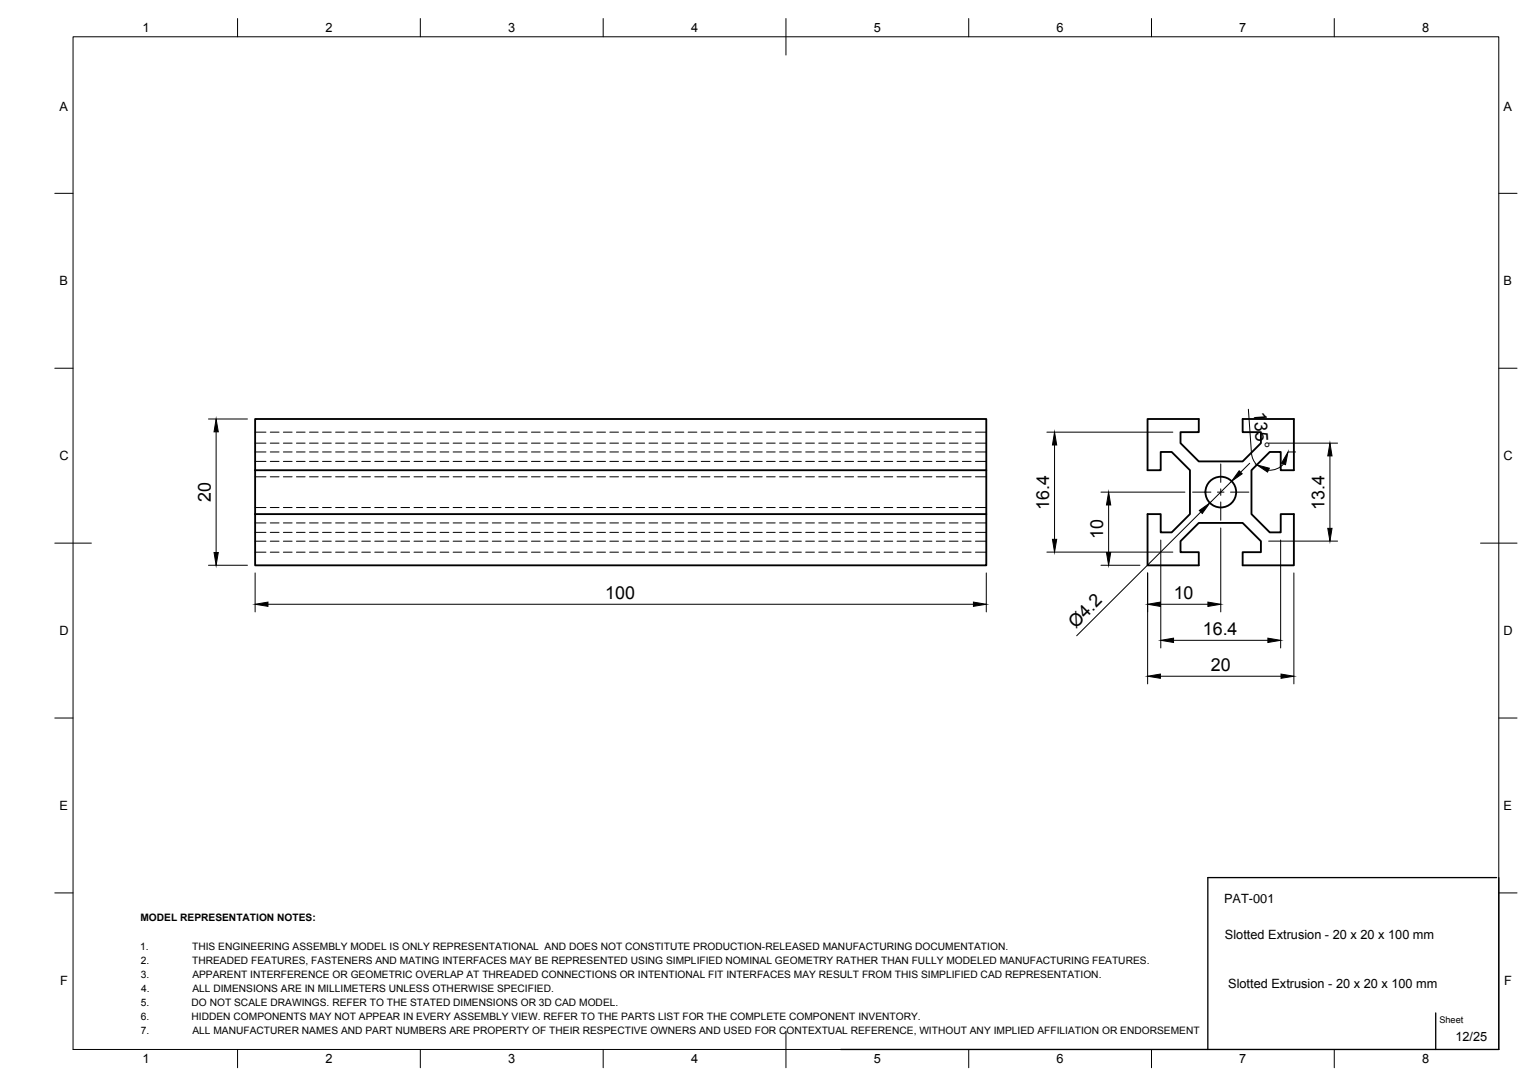
ISO-10303-21;
HEADER;
/* Generated by software containing ST-Developer
 * from STEP Tools, Inc. (www.steptools.com) 
 */

FILE_DESCRIPTION(
/* description */ ('PAT-001'),
/* implementation_level */ '2;1');

FILE_NAME(
/* name */ 'Slotted Extrusion - 20 x 20 x 100 mm.step',
/* time_stamp */ '2026-10-29T17:07:15-07:00',
/* author */ (''),
/* organization */ (''),
/* preprocessor_version */ 'ST-DEVELOPER v20.2',
/* originating_system */ 'Autodesk Translation Framework v15.17.0.0',
/* authorisation */ '');

FILE_SCHEMA (('AUTOMOTIVE_DESIGN { 1 0 10303 214 3 1 1 }'));
ENDSEC;

DATA;
#10=MECHANICAL_DESIGN_GEOMETRIC_PRESENTATION_REPRESENTATION('',(#395),#9622);
#337=SHAPE_REPRESENTATION_RELATIONSHIP('SRR','None',#9761,#362);
#362=ADVANCED_BREP_SHAPE_REPRESENTATION('',(#428),#9610);
#395=STYLED_ITEM('',(#9976),#428);
#428=MANIFOLD_SOLID_BREP('Body1',#5220);
#484=FACE_BOUND('',#1250,.T.);
#485=FACE_BOUND('',#1252,.T.);
#609=PLANE('',#5812);
#610=PLANE('',#5813);
#611=PLANE('',#5814);
#612=PLANE('',#5815);
#613=PLANE('',#5816);
#614=PLANE('',#5817);
#615=PLANE('',#5818);
#616=PLANE('',#5819);
#617=PLANE('',#5820);
#618=PLANE('',#5821);
#619=PLANE('',#5822);
#620=PLANE('',#5823);
#621=PLANE('',#5824);
#622=PLANE('',#5825);
#623=PLANE('',#5826);
#624=PLANE('',#5827);
#625=PLANE('',#5828);
#626=PLANE('',#5829);
#627=PLANE('',#5830);
#628=PLANE('',#5831);
#629=PLANE('',#5832);
#630=PLANE('',#5833);
#631=PLANE('',#5834);
#632=PLANE('',#5835);
#633=PLANE('',#5836);
#634=PLANE('',#5837);
#635=PLANE('',#5838);
#636=PLANE('',#5839);
#637=PLANE('',#5840);
#638=PLANE('',#5841);
#639=PLANE('',#5842);
#640=PLANE('',#5843);
#641=PLANE('',#5844);
#642=PLANE('',#5845);
#643=PLANE('',#5846);
#644=PLANE('',#5847);
#645=PLANE('',#5851);
#646=PLANE('',#5852);
#647=PLANE('',#5853);
#648=PLANE('',#5854);
#649=PLANE('',#5855);
#650=PLANE('',#5856);
#651=PLANE('',#5857);
#652=PLANE('',#5858);
#653=PLANE('',#5859);
#654=PLANE('',#5860);
#861=FACE_OUTER_BOUND('',#1204,.T.);
#862=FACE_OUTER_BOUND('',#1205,.T.);
#863=FACE_OUTER_BOUND('',#1206,.T.);
#864=FACE_OUTER_BOUND('',#1207,.T.);
#865=FACE_OUTER_BOUND('',#1208,.T.);
#866=FACE_OUTER_BOUND('',#1209,.T.);
#867=FACE_OUTER_BOUND('',#1210,.T.);
#868=FACE_OUTER_BOUND('',#1211,.T.);
#869=FACE_OUTER_BOUND('',#1212,.T.);
#870=FACE_OUTER_BOUND('',#1213,.T.);
#871=FACE_OUTER_BOUND('',#1214,.T.);
#872=FACE_OUTER_BOUND('',#1215,.T.);
#873=FACE_OUTER_BOUND('',#1216,.T.);
#874=FACE_OUTER_BOUND('',#1217,.T.);
#875=FACE_OUTER_BOUND('',#1218,.T.);
#876=FACE_OUTER_BOUND('',#1219,.T.);
#877=FACE_OUTER_BOUND('',#1220,.T.);
#878=FACE_OUTER_BOUND('',#1221,.T.);
#879=FACE_OUTER_BOUND('',#1222,.T.);
#880=FACE_OUTER_BOUND('',#1223,.T.);
#881=FACE_OUTER_BOUND('',#1224,.T.);
#882=FACE_OUTER_BOUND('',#1225,.T.);
#883=FACE_OUTER_BOUND('',#1226,.T.);
#884=FACE_OUTER_BOUND('',#1227,.T.);
#885=FACE_OUTER_BOUND('',#1228,.T.);
#886=FACE_OUTER_BOUND('',#1229,.T.);
#887=FACE_OUTER_BOUND('',#1230,.T.);
#888=FACE_OUTER_BOUND('',#1231,.T.);
#889=FACE_OUTER_BOUND('',#1232,.T.);
#890=FACE_OUTER_BOUND('',#1233,.T.);
#891=FACE_OUTER_BOUND('',#1234,.T.);
#892=FACE_OUTER_BOUND('',#1235,.T.);
#893=FACE_OUTER_BOUND('',#1236,.T.);
#894=FACE_OUTER_BOUND('',#1237,.T.);
#895=FACE_OUTER_BOUND('',#1238,.T.);
#896=FACE_OUTER_BOUND('',#1239,.T.);
#897=FACE_OUTER_BOUND('',#1240,.T.);
#898=FACE_OUTER_BOUND('',#1241,.T.);
#899=FACE_OUTER_BOUND('',#1242,.T.);
#900=FACE_OUTER_BOUND('',#1243,.T.);
#901=FACE_OUTER_BOUND('',#1244,.T.);
#902=FACE_OUTER_BOUND('',#1245,.T.);
#903=FACE_OUTER_BOUND('',#1246,.T.);
#904=FACE_OUTER_BOUND('',#1247,.T.);
#905=FACE_OUTER_BOUND('',#1248,.T.);
#906=FACE_OUTER_BOUND('',#1249,.T.);
#907=FACE_OUTER_BOUND('',#1251,.T.);
#1204=EDGE_LOOP('',(#4131,#4132,#4133,#4134));
#1205=EDGE_LOOP('',(#4135,#4136,#4137,#4138));
#1206=EDGE_LOOP('',(#4139,#4140,#4141,#4142));
#1207=EDGE_LOOP('',(#4143,#4144,#4145,#4146));
#1208=EDGE_LOOP('',(#4147,#4148,#4149,#4150));
#1209=EDGE_LOOP('',(#4151,#4152,#4153,#4154));
#1210=EDGE_LOOP('',(#4155,#4156,#4157,#4158));
#1211=EDGE_LOOP('',(#4159,#4160,#4161,#4162));
#1212=EDGE_LOOP('',(#4163,#4164,#4165,#4166));
#1213=EDGE_LOOP('',(#4167,#4168,#4169,#4170));
#1214=EDGE_LOOP('',(#4171,#4172,#4173,#4174));
#1215=EDGE_LOOP('',(#4175,#4176,#4177,#4178));
#1216=EDGE_LOOP('',(#4179,#4180,#4181,#4182));
#1217=EDGE_LOOP('',(#4183,#4184,#4185,#4186));
#1218=EDGE_LOOP('',(#4187,#4188,#4189,#4190));
#1219=EDGE_LOOP('',(#4191,#4192,#4193,#4194));
#1220=EDGE_LOOP('',(#4195,#4196,#4197,#4198));
#1221=EDGE_LOOP('',(#4199,#4200,#4201,#4202));
#1222=EDGE_LOOP('',(#4203,#4204,#4205,#4206));
#1223=EDGE_LOOP('',(#4207,#4208,#4209,#4210));
#1224=EDGE_LOOP('',(#4211,#4212,#4213,#4214));
#1225=EDGE_LOOP('',(#4215,#4216,#4217,#4218));
#1226=EDGE_LOOP('',(#4219,#4220,#4221,#4222));
#1227=EDGE_LOOP('',(#4223,#4224,#4225,#4226));
#1228=EDGE_LOOP('',(#4227,#4228,#4229,#4230));
#1229=EDGE_LOOP('',(#4231,#4232,#4233,#4234));
#1230=EDGE_LOOP('',(#4235,#4236,#4237,#4238));
#1231=EDGE_LOOP('',(#4239,#4240,#4241,#4242));
#1232=EDGE_LOOP('',(#4243,#4244,#4245,#4246));
#1233=EDGE_LOOP('',(#4247,#4248,#4249,#4250));
#1234=EDGE_LOOP('',(#4251,#4252,#4253,#4254));
#1235=EDGE_LOOP('',(#4255,#4256,#4257,#4258));
#1236=EDGE_LOOP('',(#4259,#4260,#4261,#4262));
#1237=EDGE_LOOP('',(#4263,#4264,#4265,#4266));
#1238=EDGE_LOOP('',(#4267,#4268,#4269,#4270));
#1239=EDGE_LOOP('',(#4271,#4272,#4273,#4274));
#1240=EDGE_LOOP('',(#4275,#4276,#4277,#4278));
#1241=EDGE_LOOP('',(#4279,#4280,#4281,#4282));
#1242=EDGE_LOOP('',(#4283,#4284,#4285,#4286));
#1243=EDGE_LOOP('',(#4287,#4288,#4289,#4290));
#1244=EDGE_LOOP('',(#4291,#4292,#4293,#4294));
#1245=EDGE_LOOP('',(#4295,#4296,#4297,#4298));
#1246=EDGE_LOOP('',(#4299,#4300,#4301,#4302));
#1247=EDGE_LOOP('',(#4303,#4304,#4305,#4306));
#1248=EDGE_LOOP('',(#4307,#4308,#4309,#4310));
#1249=EDGE_LOOP('',(#4311,#4312,#4313,#4314,#4315,#4316,#4317,#4318,#4319,
#4320,#4321,#4322,#4323,#4324,#4325,#4326,#4327,#4328,#4329,#4330,#4331,
#4332,#4333,#4334,#4335,#4336,#4337,#4338,#4339,#4340,#4341,#4342,#4343,
#4344,#4345,#4346,#4347,#4348,#4349,#4350,#4351,#4352,#4353,#4354));
#1250=EDGE_LOOP('',(#4355));
#1251=EDGE_LOOP('',(#4356,#4357,#4358,#4359,#4360,#4361,#4362,#4363,#4364,
#4365,#4366,#4367,#4368,#4369,#4370,#4371,#4372,#4373,#4374,#4375,#4376,
#4377,#4378,#4379,#4380,#4381,#4382,#4383,#4384,#4385,#4386,#4387,#4388,
#4389,#4390,#4391,#4392,#4393,#4394,#4395,#4396,#4397,#4398,#4399));
#1252=EDGE_LOOP('',(#4400));
#1553=LINE('',#8739,#1958);
#1554=LINE('',#8741,#1959);
#1555=LINE('',#8743,#1960);
#1556=LINE('',#8744,#1961);
#1557=LINE('',#8747,#1962);
#1558=LINE('',#8749,#1963);
#1559=LINE('',#8750,#1964);
#1560=LINE('',#8753,#1965);
#1561=LINE('',#8755,#1966);
#1562=LINE('',#8756,#1967);
#1563=LINE('',#8759,#1968);
#1564=LINE('',#8761,#1969);
#1565=LINE('',#8762,#1970);
#1566=LINE('',#8765,#1971);
#1567=LINE('',#8767,#1972);
#1568=LINE('',#8768,#1973);
#1569=LINE('',#8771,#1974);
#1570=LINE('',#8773,#1975);
#1571=LINE('',#8774,#1976);
#1572=LINE('',#8777,#1977);
#1573=LINE('',#8779,#1978);
#1574=LINE('',#8780,#1979);
#1575=LINE('',#8783,#1980);
#1576=LINE('',#8785,#1981);
#1577=LINE('',#8786,#1982);
#1578=LINE('',#8789,#1983);
#1579=LINE('',#8791,#1984);
#1580=LINE('',#8792,#1985);
#1581=LINE('',#8796,#1986);
#1582=LINE('',#8798,#1987);
#1583=LINE('',#8800,#1988);
#1584=LINE('',#8801,#1989);
#1585=LINE('',#8804,#1990);
#1586=LINE('',#8806,#1991);
#1587=LINE('',#8807,#1992);
#1588=LINE('',#8810,#1993);
#1589=LINE('',#8812,#1994);
#1590=LINE('',#8813,#1995);
#1591=LINE('',#8816,#1996);
#1592=LINE('',#8818,#1997);
#1593=LINE('',#8819,#1998);
#1594=LINE('',#8822,#1999);
#1595=LINE('',#8824,#2000);
#1596=LINE('',#8825,#2001);
#1597=LINE('',#8828,#2002);
#1598=LINE('',#8830,#2003);
#1599=LINE('',#8831,#2004);
#1600=LINE('',#8834,#2005);
#1601=LINE('',#8836,#2006);
#1602=LINE('',#8837,#2007);
#1603=LINE('',#8840,#2008);
#1604=LINE('',#8842,#2009);
#1605=LINE('',#8843,#2010);
#1606=LINE('',#8846,#2011);
#1607=LINE('',#8848,#2012);
#1608=LINE('',#8849,#2013);
#1609=LINE('',#8853,#2014);
#1610=LINE('',#8855,#2015);
#1611=LINE('',#8857,#2016);
#1612=LINE('',#8858,#2017);
#1613=LINE('',#8861,#2018);
#1614=LINE('',#8863,#2019);
#1615=LINE('',#8864,#2020);
#1616=LINE('',#8867,#2021);
#1617=LINE('',#8869,#2022);
#1618=LINE('',#8870,#2023);
#1619=LINE('',#8873,#2024);
#1620=LINE('',#8875,#2025);
#1621=LINE('',#8876,#2026);
#1622=LINE('',#8879,#2027);
#1623=LINE('',#8881,#2028);
#1624=LINE('',#8882,#2029);
#1625=LINE('',#8885,#2030);
#1626=LINE('',#8887,#2031);
#1627=LINE('',#8888,#2032);
#1628=LINE('',#8891,#2033);
#1629=LINE('',#8893,#2034);
#1630=LINE('',#8894,#2035);
#1631=LINE('',#8897,#2036);
#1632=LINE('',#8899,#2037);
#1633=LINE('',#8900,#2038);
#1634=LINE('',#8903,#2039);
#1635=LINE('',#8905,#2040);
#1636=LINE('',#8906,#2041);
#1637=LINE('',#8910,#2042);
#1638=LINE('',#8912,#2043);
#1639=LINE('',#8914,#2044);
#1640=LINE('',#8915,#2045);
#1641=LINE('',#8918,#2046);
#1642=LINE('',#8920,#2047);
#1643=LINE('',#8921,#2048);
#1644=LINE('',#8924,#2049);
#1645=LINE('',#8926,#2050);
#1646=LINE('',#8927,#2051);
#1647=LINE('',#8930,#2052);
#1648=LINE('',#8932,#2053);
#1649=LINE('',#8933,#2054);
#1650=LINE('',#8936,#2055);
#1651=LINE('',#8938,#2056);
#1652=LINE('',#8939,#2057);
#1653=LINE('',#8942,#2058);
#1654=LINE('',#8944,#2059);
#1655=LINE('',#8945,#2060);
#1656=LINE('',#8948,#2061);
#1657=LINE('',#8950,#2062);
#1658=LINE('',#8951,#2063);
#1659=LINE('',#8954,#2064);
#1660=LINE('',#8956,#2065);
#1661=LINE('',#8957,#2066);
#1662=LINE('',#8960,#2067);
#1663=LINE('',#8962,#2068);
#1664=LINE('',#8963,#2069);
#1665=LINE('',#8968,#2070);
#1666=LINE('',#8972,#2071);
#1667=LINE('',#8974,#2072);
#1668=LINE('',#8975,#2073);
#1669=LINE('',#8978,#2074);
#1670=LINE('',#8980,#2075);
#1671=LINE('',#8981,#2076);
#1672=LINE('',#8983,#2077);
#1673=LINE('',#8984,#2078);
#1674=LINE('',#8987,#2079);
#1675=LINE('',#8989,#2080);
#1676=LINE('',#8990,#2081);
#1677=LINE('',#8992,#2082);
#1678=LINE('',#8993,#2083);
#1679=LINE('',#8996,#2084);
#1680=LINE('',#8998,#2085);
#1681=LINE('',#8999,#2086);
#1682=LINE('',#9001,#2087);
#1683=LINE('',#9002,#2088);
#1684=LINE('',#9004,#2089);
#1685=LINE('',#9005,#2090);
#1958=VECTOR('',#6870,1.);
#1959=VECTOR('',#6871,1.);
#1960=VECTOR('',#6872,1.);
#1961=VECTOR('',#6873,1.);
#1962=VECTOR('',#6876,1.);
#1963=VECTOR('',#6877,1.);
#1964=VECTOR('',#6878,1.);
#1965=VECTOR('',#6881,1.);
#1966=VECTOR('',#6882,1.);
#1967=VECTOR('',#6883,1.);
#1968=VECTOR('',#6886,1.);
#1969=VECTOR('',#6887,1.);
#1970=VECTOR('',#6888,1.);
#1971=VECTOR('',#6891,1.);
#1972=VECTOR('',#6892,1.);
#1973=VECTOR('',#6893,1.);
#1974=VECTOR('',#6896,1.);
#1975=VECTOR('',#6897,1.);
#1976=VECTOR('',#6898,1.);
#1977=VECTOR('',#6901,1.);
#1978=VECTOR('',#6902,1.);
#1979=VECTOR('',#6903,1.);
#1980=VECTOR('',#6906,1.);
#1981=VECTOR('',#6907,1.);
#1982=VECTOR('',#6908,1.);
#1983=VECTOR('',#6911,1.);
#1984=VECTOR('',#6912,1.);
#1985=VECTOR('',#6913,1.);
#1986=VECTOR('',#6916,1.);
#1987=VECTOR('',#6917,1.);
#1988=VECTOR('',#6918,1.);
#1989=VECTOR('',#6919,1.);
#1990=VECTOR('',#6922,1.);
#1991=VECTOR('',#6923,1.);
#1992=VECTOR('',#6924,1.);
#1993=VECTOR('',#6927,1.);
#1994=VECTOR('',#6928,1.);
#1995=VECTOR('',#6929,1.);
#1996=VECTOR('',#6932,1.);
#1997=VECTOR('',#6933,1.);
#1998=VECTOR('',#6934,1.);
#1999=VECTOR('',#6937,1.);
#2000=VECTOR('',#6938,1.);
#2001=VECTOR('',#6939,1.);
#2002=VECTOR('',#6942,1.);
#2003=VECTOR('',#6943,1.);
#2004=VECTOR('',#6944,1.);
#2005=VECTOR('',#6947,1.);
#2006=VECTOR('',#6948,1.);
#2007=VECTOR('',#6949,1.);
#2008=VECTOR('',#6952,1.);
#2009=VECTOR('',#6953,1.);
#2010=VECTOR('',#6954,1.);
#2011=VECTOR('',#6957,1.);
#2012=VECTOR('',#6958,1.);
#2013=VECTOR('',#6959,1.);
#2014=VECTOR('',#6962,1.);
#2015=VECTOR('',#6963,1.);
#2016=VECTOR('',#6964,1.);
#2017=VECTOR('',#6965,1.);
#2018=VECTOR('',#6968,1.);
#2019=VECTOR('',#6969,1.);
#2020=VECTOR('',#6970,1.);
#2021=VECTOR('',#6973,1.);
#2022=VECTOR('',#6974,1.);
#2023=VECTOR('',#6975,1.);
#2024=VECTOR('',#6978,1.);
#2025=VECTOR('',#6979,1.);
#2026=VECTOR('',#6980,1.);
#2027=VECTOR('',#6983,1.);
#2028=VECTOR('',#6984,1.);
#2029=VECTOR('',#6985,1.);
#2030=VECTOR('',#6988,1.);
#2031=VECTOR('',#6989,1.);
#2032=VECTOR('',#6990,1.);
#2033=VECTOR('',#6993,1.);
#2034=VECTOR('',#6994,1.);
#2035=VECTOR('',#6995,1.);
#2036=VECTOR('',#6998,1.);
#2037=VECTOR('',#6999,1.);
#2038=VECTOR('',#7000,1.);
#2039=VECTOR('',#7003,1.);
#2040=VECTOR('',#7004,1.);
#2041=VECTOR('',#7005,1.);
#2042=VECTOR('',#7008,1.);
#2043=VECTOR('',#7009,1.);
#2044=VECTOR('',#7010,1.);
#2045=VECTOR('',#7011,1.);
#2046=VECTOR('',#7014,1.);
#2047=VECTOR('',#7015,1.);
#2048=VECTOR('',#7016,1.);
#2049=VECTOR('',#7019,1.);
#2050=VECTOR('',#7020,1.);
#2051=VECTOR('',#7021,1.);
#2052=VECTOR('',#7024,1.);
#2053=VECTOR('',#7025,1.);
#2054=VECTOR('',#7026,1.);
#2055=VECTOR('',#7029,1.);
#2056=VECTOR('',#7030,1.);
#2057=VECTOR('',#7031,1.);
#2058=VECTOR('',#7034,1.);
#2059=VECTOR('',#7035,1.);
#2060=VECTOR('',#7036,1.);
#2061=VECTOR('',#7039,1.);
#2062=VECTOR('',#7040,1.);
#2063=VECTOR('',#7041,1.);
#2064=VECTOR('',#7044,1.);
#2065=VECTOR('',#7045,1.);
#2066=VECTOR('',#7046,1.);
#2067=VECTOR('',#7049,1.);
#2068=VECTOR('',#7050,1.);
#2069=VECTOR('',#7051,1.);
#2070=VECTOR('',#7056,0.21);
#2071=VECTOR('',#7061,1.);
#2072=VECTOR('',#7062,1.);
#2073=VECTOR('',#7063,1.);
#2074=VECTOR('',#7066,1.);
#2075=VECTOR('',#7067,1.);
#2076=VECTOR('',#7068,1.);
#2077=VECTOR('',#7071,1.);
#2078=VECTOR('',#7072,1.);
#2079=VECTOR('',#7075,1.);
#2080=VECTOR('',#7076,1.);
#2081=VECTOR('',#7077,1.);
#2082=VECTOR('',#7080,1.);
#2083=VECTOR('',#7081,1.);
#2084=VECTOR('',#7084,1.);
#2085=VECTOR('',#7085,1.);
#2086=VECTOR('',#7086,1.);
#2087=VECTOR('',#7089,1.);
#2088=VECTOR('',#7090,1.);
#2089=VECTOR('',#7093,1.);
#2090=VECTOR('',#7094,1.);
#2342=CIRCLE('',#5849,0.21);
#2343=CIRCLE('',#5850,0.21);
#2634=VERTEX_POINT('',#8737);
#2635=VERTEX_POINT('',#8738);
#2636=VERTEX_POINT('',#8740);
#2637=VERTEX_POINT('',#8742);
#2638=VERTEX_POINT('',#8746);
#2639=VERTEX_POINT('',#8748);
#2640=VERTEX_POINT('',#8752);
#2641=VERTEX_POINT('',#8754);
#2642=VERTEX_POINT('',#8758);
#2643=VERTEX_POINT('',#8760);
#2644=VERTEX_POINT('',#8764);
#2645=VERTEX_POINT('',#8766);
#2646=VERTEX_POINT('',#8770);
#2647=VERTEX_POINT('',#8772);
#2648=VERTEX_POINT('',#8776);
#2649=VERTEX_POINT('',#8778);
#2650=VERTEX_POINT('',#8782);
#2651=VERTEX_POINT('',#8784);
#2652=VERTEX_POINT('',#8788);
#2653=VERTEX_POINT('',#8790);
#2654=VERTEX_POINT('',#8794);
#2655=VERTEX_POINT('',#8795);
#2656=VERTEX_POINT('',#8797);
#2657=VERTEX_POINT('',#8799);
#2658=VERTEX_POINT('',#8803);
#2659=VERTEX_POINT('',#8805);
#2660=VERTEX_POINT('',#8809);
#2661=VERTEX_POINT('',#8811);
#2662=VERTEX_POINT('',#8815);
#2663=VERTEX_POINT('',#8817);
#2664=VERTEX_POINT('',#8821);
#2665=VERTEX_POINT('',#8823);
#2666=VERTEX_POINT('',#8827);
#2667=VERTEX_POINT('',#8829);
#2668=VERTEX_POINT('',#8833);
#2669=VERTEX_POINT('',#8835);
#2670=VERTEX_POINT('',#8839);
#2671=VERTEX_POINT('',#8841);
#2672=VERTEX_POINT('',#8845);
#2673=VERTEX_POINT('',#8847);
#2674=VERTEX_POINT('',#8851);
#2675=VERTEX_POINT('',#8852);
#2676=VERTEX_POINT('',#8854);
#2677=VERTEX_POINT('',#8856);
#2678=VERTEX_POINT('',#8860);
#2679=VERTEX_POINT('',#8862);
#2680=VERTEX_POINT('',#8866);
#2681=VERTEX_POINT('',#8868);
#2682=VERTEX_POINT('',#8872);
#2683=VERTEX_POINT('',#8874);
#2684=VERTEX_POINT('',#8878);
#2685=VERTEX_POINT('',#8880);
#2686=VERTEX_POINT('',#8884);
#2687=VERTEX_POINT('',#8886);
#2688=VERTEX_POINT('',#8890);
#2689=VERTEX_POINT('',#8892);
#2690=VERTEX_POINT('',#8896);
#2691=VERTEX_POINT('',#8898);
#2692=VERTEX_POINT('',#8902);
#2693=VERTEX_POINT('',#8904);
#2694=VERTEX_POINT('',#8908);
#2695=VERTEX_POINT('',#8909);
#2696=VERTEX_POINT('',#8911);
#2697=VERTEX_POINT('',#8913);
#2698=VERTEX_POINT('',#8917);
#2699=VERTEX_POINT('',#8919);
#2700=VERTEX_POINT('',#8923);
#2701=VERTEX_POINT('',#8925);
#2702=VERTEX_POINT('',#8929);
#2703=VERTEX_POINT('',#8931);
#2704=VERTEX_POINT('',#8935);
#2705=VERTEX_POINT('',#8937);
#2706=VERTEX_POINT('',#8941);
#2707=VERTEX_POINT('',#8943);
#2708=VERTEX_POINT('',#8947);
#2709=VERTEX_POINT('',#8949);
#2710=VERTEX_POINT('',#8953);
#2711=VERTEX_POINT('',#8955);
#2712=VERTEX_POINT('',#8959);
#2713=VERTEX_POINT('',#8961);
#2714=VERTEX_POINT('',#8965);
#2715=VERTEX_POINT('',#8967);
#2716=VERTEX_POINT('',#8971);
#2717=VERTEX_POINT('',#8973);
#2718=VERTEX_POINT('',#8977);
#2719=VERTEX_POINT('',#8979);
#2720=VERTEX_POINT('',#8986);
#2721=VERTEX_POINT('',#8988);
#2722=VERTEX_POINT('',#8995);
#2723=VERTEX_POINT('',#8997);
#3169=EDGE_CURVE('',#2634,#2635,#1553,.T.);
#3170=EDGE_CURVE('',#2634,#2636,#1554,.T.);
#3171=EDGE_CURVE('',#2637,#2636,#1555,.T.);
#3172=EDGE_CURVE('',#2635,#2637,#1556,.T.);
#3173=EDGE_CURVE('',#2638,#2634,#1557,.T.);
#3174=EDGE_CURVE('',#2638,#2639,#1558,.T.);
#3175=EDGE_CURVE('',#2636,#2639,#1559,.T.);
#3176=EDGE_CURVE('',#2640,#2638,#1560,.T.);
#3177=EDGE_CURVE('',#2640,#2641,#1561,.T.);
#3178=EDGE_CURVE('',#2639,#2641,#1562,.T.);
#3179=EDGE_CURVE('',#2642,#2640,#1563,.T.);
#3180=EDGE_CURVE('',#2642,#2643,#1564,.T.);
#3181=EDGE_CURVE('',#2641,#2643,#1565,.T.);
#3182=EDGE_CURVE('',#2644,#2642,#1566,.T.);
#3183=EDGE_CURVE('',#2644,#2645,#1567,.T.);
#3184=EDGE_CURVE('',#2643,#2645,#1568,.T.);
#3185=EDGE_CURVE('',#2646,#2644,#1569,.T.);
#3186=EDGE_CURVE('',#2646,#2647,#1570,.T.);
#3187=EDGE_CURVE('',#2645,#2647,#1571,.T.);
#3188=EDGE_CURVE('',#2648,#2646,#1572,.T.);
#3189=EDGE_CURVE('',#2648,#2649,#1573,.T.);
#3190=EDGE_CURVE('',#2647,#2649,#1574,.T.);
#3191=EDGE_CURVE('',#2650,#2648,#1575,.T.);
#3192=EDGE_CURVE('',#2650,#2651,#1576,.T.);
#3193=EDGE_CURVE('',#2649,#2651,#1577,.T.);
#3194=EDGE_CURVE('',#2652,#2650,#1578,.T.);
#3195=EDGE_CURVE('',#2653,#2652,#1579,.T.);
#3196=EDGE_CURVE('',#2651,#2653,#1580,.T.);
#3197=EDGE_CURVE('',#2654,#2655,#1581,.T.);
#3198=EDGE_CURVE('',#2654,#2656,#1582,.T.);
#3199=EDGE_CURVE('',#2657,#2656,#1583,.T.);
#3200=EDGE_CURVE('',#2655,#2657,#1584,.T.);
#3201=EDGE_CURVE('',#2658,#2654,#1585,.T.);
#3202=EDGE_CURVE('',#2658,#2659,#1586,.T.);
#3203=EDGE_CURVE('',#2656,#2659,#1587,.T.);
#3204=EDGE_CURVE('',#2660,#2658,#1588,.T.);
#3205=EDGE_CURVE('',#2660,#2661,#1589,.T.);
#3206=EDGE_CURVE('',#2659,#2661,#1590,.T.);
#3207=EDGE_CURVE('',#2662,#2660,#1591,.T.);
#3208=EDGE_CURVE('',#2662,#2663,#1592,.T.);
#3209=EDGE_CURVE('',#2661,#2663,#1593,.T.);
#3210=EDGE_CURVE('',#2664,#2662,#1594,.T.);
#3211=EDGE_CURVE('',#2664,#2665,#1595,.T.);
#3212=EDGE_CURVE('',#2663,#2665,#1596,.T.);
#3213=EDGE_CURVE('',#2666,#2664,#1597,.T.);
#3214=EDGE_CURVE('',#2666,#2667,#1598,.T.);
#3215=EDGE_CURVE('',#2665,#2667,#1599,.T.);
#3216=EDGE_CURVE('',#2668,#2666,#1600,.T.);
#3217=EDGE_CURVE('',#2668,#2669,#1601,.T.);
#3218=EDGE_CURVE('',#2667,#2669,#1602,.T.);
#3219=EDGE_CURVE('',#2670,#2668,#1603,.T.);
#3220=EDGE_CURVE('',#2670,#2671,#1604,.T.);
#3221=EDGE_CURVE('',#2669,#2671,#1605,.T.);
#3222=EDGE_CURVE('',#2672,#2670,#1606,.T.);
#3223=EDGE_CURVE('',#2673,#2672,#1607,.T.);
#3224=EDGE_CURVE('',#2671,#2673,#1608,.T.);
#3225=EDGE_CURVE('',#2674,#2675,#1609,.T.);
#3226=EDGE_CURVE('',#2674,#2676,#1610,.T.);
#3227=EDGE_CURVE('',#2677,#2676,#1611,.T.);
#3228=EDGE_CURVE('',#2675,#2677,#1612,.T.);
#3229=EDGE_CURVE('',#2678,#2674,#1613,.T.);
#3230=EDGE_CURVE('',#2678,#2679,#1614,.T.);
#3231=EDGE_CURVE('',#2676,#2679,#1615,.T.);
#3232=EDGE_CURVE('',#2680,#2678,#1616,.T.);
#3233=EDGE_CURVE('',#2680,#2681,#1617,.T.);
#3234=EDGE_CURVE('',#2679,#2681,#1618,.T.);
#3235=EDGE_CURVE('',#2682,#2680,#1619,.T.);
#3236=EDGE_CURVE('',#2682,#2683,#1620,.T.);
#3237=EDGE_CURVE('',#2681,#2683,#1621,.T.);
#3238=EDGE_CURVE('',#2684,#2682,#1622,.T.);
#3239=EDGE_CURVE('',#2684,#2685,#1623,.T.);
#3240=EDGE_CURVE('',#2683,#2685,#1624,.T.);
#3241=EDGE_CURVE('',#2686,#2684,#1625,.T.);
#3242=EDGE_CURVE('',#2686,#2687,#1626,.T.);
#3243=EDGE_CURVE('',#2685,#2687,#1627,.T.);
#3244=EDGE_CURVE('',#2688,#2686,#1628,.T.);
#3245=EDGE_CURVE('',#2688,#2689,#1629,.T.);
#3246=EDGE_CURVE('',#2687,#2689,#1630,.T.);
#3247=EDGE_CURVE('',#2690,#2688,#1631,.T.);
#3248=EDGE_CURVE('',#2690,#2691,#1632,.T.);
#3249=EDGE_CURVE('',#2689,#2691,#1633,.T.);
#3250=EDGE_CURVE('',#2692,#2690,#1634,.T.);
#3251=EDGE_CURVE('',#2693,#2692,#1635,.T.);
#3252=EDGE_CURVE('',#2691,#2693,#1636,.T.);
#3253=EDGE_CURVE('',#2694,#2695,#1637,.T.);
#3254=EDGE_CURVE('',#2694,#2696,#1638,.T.);
#3255=EDGE_CURVE('',#2697,#2696,#1639,.T.);
#3256=EDGE_CURVE('',#2695,#2697,#1640,.T.);
#3257=EDGE_CURVE('',#2698,#2694,#1641,.T.);
#3258=EDGE_CURVE('',#2698,#2699,#1642,.T.);
#3259=EDGE_CURVE('',#2696,#2699,#1643,.T.);
#3260=EDGE_CURVE('',#2700,#2698,#1644,.T.);
#3261=EDGE_CURVE('',#2700,#2701,#1645,.T.);
#3262=EDGE_CURVE('',#2699,#2701,#1646,.T.);
#3263=EDGE_CURVE('',#2702,#2700,#1647,.T.);
#3264=EDGE_CURVE('',#2702,#2703,#1648,.T.);
#3265=EDGE_CURVE('',#2701,#2703,#1649,.T.);
#3266=EDGE_CURVE('',#2704,#2702,#1650,.T.);
#3267=EDGE_CURVE('',#2704,#2705,#1651,.T.);
#3268=EDGE_CURVE('',#2703,#2705,#1652,.T.);
#3269=EDGE_CURVE('',#2706,#2704,#1653,.T.);
#3270=EDGE_CURVE('',#2706,#2707,#1654,.T.);
#3271=EDGE_CURVE('',#2705,#2707,#1655,.T.);
#3272=EDGE_CURVE('',#2708,#2706,#1656,.T.);
#3273=EDGE_CURVE('',#2708,#2709,#1657,.T.);
#3274=EDGE_CURVE('',#2707,#2709,#1658,.T.);
#3275=EDGE_CURVE('',#2710,#2708,#1659,.T.);
#3276=EDGE_CURVE('',#2710,#2711,#1660,.T.);
#3277=EDGE_CURVE('',#2709,#2711,#1661,.T.);
#3278=EDGE_CURVE('',#2712,#2710,#1662,.T.);
#3279=EDGE_CURVE('',#2713,#2712,#1663,.T.);
#3280=EDGE_CURVE('',#2711,#2713,#1664,.T.);
#3281=EDGE_CURVE('',#2714,#2714,#2342,.T.);
#3282=EDGE_CURVE('',#2714,#2715,#1665,.T.);
#3283=EDGE_CURVE('',#2715,#2715,#2343,.T.);
#3284=EDGE_CURVE('',#2652,#2716,#1666,.T.);
#3285=EDGE_CURVE('',#2716,#2717,#1667,.T.);
#3286=EDGE_CURVE('',#2653,#2717,#1668,.T.);
#3287=EDGE_CURVE('',#2718,#2637,#1669,.T.);
#3288=EDGE_CURVE('',#2719,#2718,#1670,.T.);
#3289=EDGE_CURVE('',#2719,#2635,#1671,.T.);
#3290=EDGE_CURVE('',#2672,#2719,#1672,.T.);
#3291=EDGE_CURVE('',#2673,#2718,#1673,.T.);
#3292=EDGE_CURVE('',#2720,#2657,#1674,.T.);
#3293=EDGE_CURVE('',#2721,#2720,#1675,.T.);
#3294=EDGE_CURVE('',#2721,#2655,#1676,.T.);
#3295=EDGE_CURVE('',#2692,#2721,#1677,.T.);
#3296=EDGE_CURVE('',#2693,#2720,#1678,.T.);
#3297=EDGE_CURVE('',#2722,#2677,#1679,.T.);
#3298=EDGE_CURVE('',#2723,#2722,#1680,.T.);
#3299=EDGE_CURVE('',#2723,#2675,#1681,.T.);
#3300=EDGE_CURVE('',#2712,#2723,#1682,.T.);
#3301=EDGE_CURVE('',#2713,#2722,#1683,.T.);
#3302=EDGE_CURVE('',#2717,#2697,#1684,.T.);
#3303=EDGE_CURVE('',#2716,#2695,#1685,.T.);
#4131=ORIENTED_EDGE('',*,*,#3169,.F.);
#4132=ORIENTED_EDGE('',*,*,#3170,.T.);
#4133=ORIENTED_EDGE('',*,*,#3171,.F.);
#4134=ORIENTED_EDGE('',*,*,#3172,.F.);
#4135=ORIENTED_EDGE('',*,*,#3173,.F.);
#4136=ORIENTED_EDGE('',*,*,#3174,.T.);
#4137=ORIENTED_EDGE('',*,*,#3175,.F.);
#4138=ORIENTED_EDGE('',*,*,#3170,.F.);
#4139=ORIENTED_EDGE('',*,*,#3176,.F.);
#4140=ORIENTED_EDGE('',*,*,#3177,.T.);
#4141=ORIENTED_EDGE('',*,*,#3178,.F.);
#4142=ORIENTED_EDGE('',*,*,#3174,.F.);
#4143=ORIENTED_EDGE('',*,*,#3179,.F.);
#4144=ORIENTED_EDGE('',*,*,#3180,.T.);
#4145=ORIENTED_EDGE('',*,*,#3181,.F.);
#4146=ORIENTED_EDGE('',*,*,#3177,.F.);
#4147=ORIENTED_EDGE('',*,*,#3182,.F.);
#4148=ORIENTED_EDGE('',*,*,#3183,.T.);
#4149=ORIENTED_EDGE('',*,*,#3184,.F.);
#4150=ORIENTED_EDGE('',*,*,#3180,.F.);
#4151=ORIENTED_EDGE('',*,*,#3185,.F.);
#4152=ORIENTED_EDGE('',*,*,#3186,.T.);
#4153=ORIENTED_EDGE('',*,*,#3187,.F.);
#4154=ORIENTED_EDGE('',*,*,#3183,.F.);
#4155=ORIENTED_EDGE('',*,*,#3188,.F.);
#4156=ORIENTED_EDGE('',*,*,#3189,.T.);
#4157=ORIENTED_EDGE('',*,*,#3190,.F.);
#4158=ORIENTED_EDGE('',*,*,#3186,.F.);
#4159=ORIENTED_EDGE('',*,*,#3191,.F.);
#4160=ORIENTED_EDGE('',*,*,#3192,.T.);
#4161=ORIENTED_EDGE('',*,*,#3193,.F.);
#4162=ORIENTED_EDGE('',*,*,#3189,.F.);
#4163=ORIENTED_EDGE('',*,*,#3194,.F.);
#4164=ORIENTED_EDGE('',*,*,#3195,.F.);
#4165=ORIENTED_EDGE('',*,*,#3196,.F.);
#4166=ORIENTED_EDGE('',*,*,#3192,.F.);
#4167=ORIENTED_EDGE('',*,*,#3197,.F.);
#4168=ORIENTED_EDGE('',*,*,#3198,.T.);
#4169=ORIENTED_EDGE('',*,*,#3199,.F.);
#4170=ORIENTED_EDGE('',*,*,#3200,.F.);
#4171=ORIENTED_EDGE('',*,*,#3201,.F.);
#4172=ORIENTED_EDGE('',*,*,#3202,.T.);
#4173=ORIENTED_EDGE('',*,*,#3203,.F.);
#4174=ORIENTED_EDGE('',*,*,#3198,.F.);
#4175=ORIENTED_EDGE('',*,*,#3204,.F.);
#4176=ORIENTED_EDGE('',*,*,#3205,.T.);
#4177=ORIENTED_EDGE('',*,*,#3206,.F.);
#4178=ORIENTED_EDGE('',*,*,#3202,.F.);
#4179=ORIENTED_EDGE('',*,*,#3207,.F.);
#4180=ORIENTED_EDGE('',*,*,#3208,.T.);
#4181=ORIENTED_EDGE('',*,*,#3209,.F.);
#4182=ORIENTED_EDGE('',*,*,#3205,.F.);
#4183=ORIENTED_EDGE('',*,*,#3210,.F.);
#4184=ORIENTED_EDGE('',*,*,#3211,.T.);
#4185=ORIENTED_EDGE('',*,*,#3212,.F.);
#4186=ORIENTED_EDGE('',*,*,#3208,.F.);
#4187=ORIENTED_EDGE('',*,*,#3213,.F.);
#4188=ORIENTED_EDGE('',*,*,#3214,.T.);
#4189=ORIENTED_EDGE('',*,*,#3215,.F.);
#4190=ORIENTED_EDGE('',*,*,#3211,.F.);
#4191=ORIENTED_EDGE('',*,*,#3216,.F.);
#4192=ORIENTED_EDGE('',*,*,#3217,.T.);
#4193=ORIENTED_EDGE('',*,*,#3218,.F.);
#4194=ORIENTED_EDGE('',*,*,#3214,.F.);
#4195=ORIENTED_EDGE('',*,*,#3219,.F.);
#4196=ORIENTED_EDGE('',*,*,#3220,.T.);
#4197=ORIENTED_EDGE('',*,*,#3221,.F.);
#4198=ORIENTED_EDGE('',*,*,#3217,.F.);
#4199=ORIENTED_EDGE('',*,*,#3222,.F.);
#4200=ORIENTED_EDGE('',*,*,#3223,.F.);
#4201=ORIENTED_EDGE('',*,*,#3224,.F.);
#4202=ORIENTED_EDGE('',*,*,#3220,.F.);
#4203=ORIENTED_EDGE('',*,*,#3225,.F.);
#4204=ORIENTED_EDGE('',*,*,#3226,.T.);
#4205=ORIENTED_EDGE('',*,*,#3227,.F.);
#4206=ORIENTED_EDGE('',*,*,#3228,.F.);
#4207=ORIENTED_EDGE('',*,*,#3229,.F.);
#4208=ORIENTED_EDGE('',*,*,#3230,.T.);
#4209=ORIENTED_EDGE('',*,*,#3231,.F.);
#4210=ORIENTED_EDGE('',*,*,#3226,.F.);
#4211=ORIENTED_EDGE('',*,*,#3232,.F.);
#4212=ORIENTED_EDGE('',*,*,#3233,.T.);
#4213=ORIENTED_EDGE('',*,*,#3234,.F.);
#4214=ORIENTED_EDGE('',*,*,#3230,.F.);
#4215=ORIENTED_EDGE('',*,*,#3235,.F.);
#4216=ORIENTED_EDGE('',*,*,#3236,.T.);
#4217=ORIENTED_EDGE('',*,*,#3237,.F.);
#4218=ORIENTED_EDGE('',*,*,#3233,.F.);
#4219=ORIENTED_EDGE('',*,*,#3238,.F.);
#4220=ORIENTED_EDGE('',*,*,#3239,.T.);
#4221=ORIENTED_EDGE('',*,*,#3240,.F.);
#4222=ORIENTED_EDGE('',*,*,#3236,.F.);
#4223=ORIENTED_EDGE('',*,*,#3241,.F.);
#4224=ORIENTED_EDGE('',*,*,#3242,.T.);
#4225=ORIENTED_EDGE('',*,*,#3243,.F.);
#4226=ORIENTED_EDGE('',*,*,#3239,.F.);
#4227=ORIENTED_EDGE('',*,*,#3244,.F.);
#4228=ORIENTED_EDGE('',*,*,#3245,.T.);
#4229=ORIENTED_EDGE('',*,*,#3246,.F.);
#4230=ORIENTED_EDGE('',*,*,#3242,.F.);
#4231=ORIENTED_EDGE('',*,*,#3247,.F.);
#4232=ORIENTED_EDGE('',*,*,#3248,.T.);
#4233=ORIENTED_EDGE('',*,*,#3249,.F.);
#4234=ORIENTED_EDGE('',*,*,#3245,.F.);
#4235=ORIENTED_EDGE('',*,*,#3250,.F.);
#4236=ORIENTED_EDGE('',*,*,#3251,.F.);
#4237=ORIENTED_EDGE('',*,*,#3252,.F.);
#4238=ORIENTED_EDGE('',*,*,#3248,.F.);
#4239=ORIENTED_EDGE('',*,*,#3253,.F.);
#4240=ORIENTED_EDGE('',*,*,#3254,.T.);
#4241=ORIENTED_EDGE('',*,*,#3255,.F.);
#4242=ORIENTED_EDGE('',*,*,#3256,.F.);
#4243=ORIENTED_EDGE('',*,*,#3257,.F.);
#4244=ORIENTED_EDGE('',*,*,#3258,.T.);
#4245=ORIENTED_EDGE('',*,*,#3259,.F.);
#4246=ORIENTED_EDGE('',*,*,#3254,.F.);
#4247=ORIENTED_EDGE('',*,*,#3260,.F.);
#4248=ORIENTED_EDGE('',*,*,#3261,.T.);
#4249=ORIENTED_EDGE('',*,*,#3262,.F.);
#4250=ORIENTED_EDGE('',*,*,#3258,.F.);
#4251=ORIENTED_EDGE('',*,*,#3263,.F.);
#4252=ORIENTED_EDGE('',*,*,#3264,.T.);
#4253=ORIENTED_EDGE('',*,*,#3265,.F.);
#4254=ORIENTED_EDGE('',*,*,#3261,.F.);
#4255=ORIENTED_EDGE('',*,*,#3266,.F.);
#4256=ORIENTED_EDGE('',*,*,#3267,.T.);
#4257=ORIENTED_EDGE('',*,*,#3268,.F.);
#4258=ORIENTED_EDGE('',*,*,#3264,.F.);
#4259=ORIENTED_EDGE('',*,*,#3269,.F.);
#4260=ORIENTED_EDGE('',*,*,#3270,.T.);
#4261=ORIENTED_EDGE('',*,*,#3271,.F.);
#4262=ORIENTED_EDGE('',*,*,#3267,.F.);
#4263=ORIENTED_EDGE('',*,*,#3272,.F.);
#4264=ORIENTED_EDGE('',*,*,#3273,.T.);
#4265=ORIENTED_EDGE('',*,*,#3274,.F.);
#4266=ORIENTED_EDGE('',*,*,#3270,.F.);
#4267=ORIENTED_EDGE('',*,*,#3275,.F.);
#4268=ORIENTED_EDGE('',*,*,#3276,.T.);
#4269=ORIENTED_EDGE('',*,*,#3277,.F.);
#4270=ORIENTED_EDGE('',*,*,#3273,.F.);
#4271=ORIENTED_EDGE('',*,*,#3278,.F.);
#4272=ORIENTED_EDGE('',*,*,#3279,.F.);
#4273=ORIENTED_EDGE('',*,*,#3280,.F.);
#4274=ORIENTED_EDGE('',*,*,#3276,.F.);
#4275=ORIENTED_EDGE('',*,*,#3281,.F.);
#4276=ORIENTED_EDGE('',*,*,#3282,.T.);
#4277=ORIENTED_EDGE('',*,*,#3283,.F.);
#4278=ORIENTED_EDGE('',*,*,#3282,.F.);
#4279=ORIENTED_EDGE('',*,*,#3195,.T.);
#4280=ORIENTED_EDGE('',*,*,#3284,.T.);
#4281=ORIENTED_EDGE('',*,*,#3285,.T.);
#4282=ORIENTED_EDGE('',*,*,#3286,.F.);
#4283=ORIENTED_EDGE('',*,*,#3172,.T.);
#4284=ORIENTED_EDGE('',*,*,#3287,.F.);
#4285=ORIENTED_EDGE('',*,*,#3288,.F.);
#4286=ORIENTED_EDGE('',*,*,#3289,.T.);
#4287=ORIENTED_EDGE('',*,*,#3223,.T.);
#4288=ORIENTED_EDGE('',*,*,#3290,.T.);
#4289=ORIENTED_EDGE('',*,*,#3288,.T.);
#4290=ORIENTED_EDGE('',*,*,#3291,.F.);
#4291=ORIENTED_EDGE('',*,*,#3200,.T.);
#4292=ORIENTED_EDGE('',*,*,#3292,.F.);
#4293=ORIENTED_EDGE('',*,*,#3293,.F.);
#4294=ORIENTED_EDGE('',*,*,#3294,.T.);
#4295=ORIENTED_EDGE('',*,*,#3251,.T.);
#4296=ORIENTED_EDGE('',*,*,#3295,.T.);
#4297=ORIENTED_EDGE('',*,*,#3293,.T.);
#4298=ORIENTED_EDGE('',*,*,#3296,.F.);
#4299=ORIENTED_EDGE('',*,*,#3228,.T.);
#4300=ORIENTED_EDGE('',*,*,#3297,.F.);
#4301=ORIENTED_EDGE('',*,*,#3298,.F.);
#4302=ORIENTED_EDGE('',*,*,#3299,.T.);
#4303=ORIENTED_EDGE('',*,*,#3279,.T.);
#4304=ORIENTED_EDGE('',*,*,#3300,.T.);
#4305=ORIENTED_EDGE('',*,*,#3298,.T.);
#4306=ORIENTED_EDGE('',*,*,#3301,.F.);
#4307=ORIENTED_EDGE('',*,*,#3256,.T.);
#4308=ORIENTED_EDGE('',*,*,#3302,.F.);
#4309=ORIENTED_EDGE('',*,*,#3285,.F.);
#4310=ORIENTED_EDGE('',*,*,#3303,.T.);
#4311=ORIENTED_EDGE('',*,*,#3171,.T.);
#4312=ORIENTED_EDGE('',*,*,#3175,.T.);
#4313=ORIENTED_EDGE('',*,*,#3178,.T.);
#4314=ORIENTED_EDGE('',*,*,#3181,.T.);
#4315=ORIENTED_EDGE('',*,*,#3184,.T.);
#4316=ORIENTED_EDGE('',*,*,#3187,.T.);
#4317=ORIENTED_EDGE('',*,*,#3190,.T.);
#4318=ORIENTED_EDGE('',*,*,#3193,.T.);
#4319=ORIENTED_EDGE('',*,*,#3196,.T.);
#4320=ORIENTED_EDGE('',*,*,#3286,.T.);
#4321=ORIENTED_EDGE('',*,*,#3302,.T.);
#4322=ORIENTED_EDGE('',*,*,#3255,.T.);
#4323=ORIENTED_EDGE('',*,*,#3259,.T.);
#4324=ORIENTED_EDGE('',*,*,#3262,.T.);
#4325=ORIENTED_EDGE('',*,*,#3265,.T.);
#4326=ORIENTED_EDGE('',*,*,#3268,.T.);
#4327=ORIENTED_EDGE('',*,*,#3271,.T.);
#4328=ORIENTED_EDGE('',*,*,#3274,.T.);
#4329=ORIENTED_EDGE('',*,*,#3277,.T.);
#4330=ORIENTED_EDGE('',*,*,#3280,.T.);
#4331=ORIENTED_EDGE('',*,*,#3301,.T.);
#4332=ORIENTED_EDGE('',*,*,#3297,.T.);
#4333=ORIENTED_EDGE('',*,*,#3227,.T.);
#4334=ORIENTED_EDGE('',*,*,#3231,.T.);
#4335=ORIENTED_EDGE('',*,*,#3234,.T.);
#4336=ORIENTED_EDGE('',*,*,#3237,.T.);
#4337=ORIENTED_EDGE('',*,*,#3240,.T.);
#4338=ORIENTED_EDGE('',*,*,#3243,.T.);
#4339=ORIENTED_EDGE('',*,*,#3246,.T.);
#4340=ORIENTED_EDGE('',*,*,#3249,.T.);
#4341=ORIENTED_EDGE('',*,*,#3252,.T.);
#4342=ORIENTED_EDGE('',*,*,#3296,.T.);
#4343=ORIENTED_EDGE('',*,*,#3292,.T.);
#4344=ORIENTED_EDGE('',*,*,#3199,.T.);
#4345=ORIENTED_EDGE('',*,*,#3203,.T.);
#4346=ORIENTED_EDGE('',*,*,#3206,.T.);
#4347=ORIENTED_EDGE('',*,*,#3209,.T.);
#4348=ORIENTED_EDGE('',*,*,#3212,.T.);
#4349=ORIENTED_EDGE('',*,*,#3215,.T.);
#4350=ORIENTED_EDGE('',*,*,#3218,.T.);
#4351=ORIENTED_EDGE('',*,*,#3221,.T.);
#4352=ORIENTED_EDGE('',*,*,#3224,.T.);
#4353=ORIENTED_EDGE('',*,*,#3291,.T.);
#4354=ORIENTED_EDGE('',*,*,#3287,.T.);
#4355=ORIENTED_EDGE('',*,*,#3283,.T.);
#4356=ORIENTED_EDGE('',*,*,#3169,.T.);
#4357=ORIENTED_EDGE('',*,*,#3289,.F.);
#4358=ORIENTED_EDGE('',*,*,#3290,.F.);
#4359=ORIENTED_EDGE('',*,*,#3222,.T.);
#4360=ORIENTED_EDGE('',*,*,#3219,.T.);
#4361=ORIENTED_EDGE('',*,*,#3216,.T.);
#4362=ORIENTED_EDGE('',*,*,#3213,.T.);
#4363=ORIENTED_EDGE('',*,*,#3210,.T.);
#4364=ORIENTED_EDGE('',*,*,#3207,.T.);
#4365=ORIENTED_EDGE('',*,*,#3204,.T.);
#4366=ORIENTED_EDGE('',*,*,#3201,.T.);
#4367=ORIENTED_EDGE('',*,*,#3197,.T.);
#4368=ORIENTED_EDGE('',*,*,#3294,.F.);
#4369=ORIENTED_EDGE('',*,*,#3295,.F.);
#4370=ORIENTED_EDGE('',*,*,#3250,.T.);
#4371=ORIENTED_EDGE('',*,*,#3247,.T.);
#4372=ORIENTED_EDGE('',*,*,#3244,.T.);
#4373=ORIENTED_EDGE('',*,*,#3241,.T.);
#4374=ORIENTED_EDGE('',*,*,#3238,.T.);
#4375=ORIENTED_EDGE('',*,*,#3235,.T.);
#4376=ORIENTED_EDGE('',*,*,#3232,.T.);
#4377=ORIENTED_EDGE('',*,*,#3229,.T.);
#4378=ORIENTED_EDGE('',*,*,#3225,.T.);
#4379=ORIENTED_EDGE('',*,*,#3299,.F.);
#4380=ORIENTED_EDGE('',*,*,#3300,.F.);
#4381=ORIENTED_EDGE('',*,*,#3278,.T.);
#4382=ORIENTED_EDGE('',*,*,#3275,.T.);
#4383=ORIENTED_EDGE('',*,*,#3272,.T.);
#4384=ORIENTED_EDGE('',*,*,#3269,.T.);
#4385=ORIENTED_EDGE('',*,*,#3266,.T.);
#4386=ORIENTED_EDGE('',*,*,#3263,.T.);
#4387=ORIENTED_EDGE('',*,*,#3260,.T.);
#4388=ORIENTED_EDGE('',*,*,#3257,.T.);
#4389=ORIENTED_EDGE('',*,*,#3253,.T.);
#4390=ORIENTED_EDGE('',*,*,#3303,.F.);
#4391=ORIENTED_EDGE('',*,*,#3284,.F.);
#4392=ORIENTED_EDGE('',*,*,#3194,.T.);
#4393=ORIENTED_EDGE('',*,*,#3191,.T.);
#4394=ORIENTED_EDGE('',*,*,#3188,.T.);
#4395=ORIENTED_EDGE('',*,*,#3185,.T.);
#4396=ORIENTED_EDGE('',*,*,#3182,.T.);
#4397=ORIENTED_EDGE('',*,*,#3179,.T.);
#4398=ORIENTED_EDGE('',*,*,#3176,.T.);
#4399=ORIENTED_EDGE('',*,*,#3173,.T.);
#4400=ORIENTED_EDGE('',*,*,#3281,.T.);
#4870=CYLINDRICAL_SURFACE('',#5848,0.21);
#5048=ADVANCED_FACE('',(#861),#609,.F.);
#5049=ADVANCED_FACE('',(#862),#610,.F.);
#5050=ADVANCED_FACE('',(#863),#611,.F.);
#5051=ADVANCED_FACE('',(#864),#612,.F.);
#5052=ADVANCED_FACE('',(#865),#613,.F.);
#5053=ADVANCED_FACE('',(#866),#614,.F.);
#5054=ADVANCED_FACE('',(#867),#615,.F.);
#5055=ADVANCED_FACE('',(#868),#616,.F.);
#5056=ADVANCED_FACE('',(#869),#617,.F.);
#5057=ADVANCED_FACE('',(#870),#618,.F.);
#5058=ADVANCED_FACE('',(#871),#619,.F.);
#5059=ADVANCED_FACE('',(#872),#620,.F.);
#5060=ADVANCED_FACE('',(#873),#621,.F.);
#5061=ADVANCED_FACE('',(#874),#622,.F.);
#5062=ADVANCED_FACE('',(#875),#623,.F.);
#5063=ADVANCED_FACE('',(#876),#624,.F.);
#5064=ADVANCED_FACE('',(#877),#625,.F.);
#5065=ADVANCED_FACE('',(#878),#626,.F.);
#5066=ADVANCED_FACE('',(#879),#627,.F.);
#5067=ADVANCED_FACE('',(#880),#628,.F.);
#5068=ADVANCED_FACE('',(#881),#629,.F.);
#5069=ADVANCED_FACE('',(#882),#630,.F.);
#5070=ADVANCED_FACE('',(#883),#631,.F.);
#5071=ADVANCED_FACE('',(#884),#632,.F.);
#5072=ADVANCED_FACE('',(#885),#633,.F.);
#5073=ADVANCED_FACE('',(#886),#634,.F.);
#5074=ADVANCED_FACE('',(#887),#635,.F.);
#5075=ADVANCED_FACE('',(#888),#636,.F.);
#5076=ADVANCED_FACE('',(#889),#637,.F.);
#5077=ADVANCED_FACE('',(#890),#638,.F.);
#5078=ADVANCED_FACE('',(#891),#639,.F.);
#5079=ADVANCED_FACE('',(#892),#640,.F.);
#5080=ADVANCED_FACE('',(#893),#641,.F.);
#5081=ADVANCED_FACE('',(#894),#642,.F.);
#5082=ADVANCED_FACE('',(#895),#643,.F.);
#5083=ADVANCED_FACE('',(#896),#644,.F.);
#5084=ADVANCED_FACE('',(#897),#4870,.F.);
#5085=ADVANCED_FACE('',(#898),#645,.T.);
#5086=ADVANCED_FACE('',(#899),#646,.T.);
#5087=ADVANCED_FACE('',(#900),#647,.T.);
#5088=ADVANCED_FACE('',(#901),#648,.T.);
#5089=ADVANCED_FACE('',(#902),#649,.T.);
#5090=ADVANCED_FACE('',(#903),#650,.T.);
#5091=ADVANCED_FACE('',(#904),#651,.T.);
#5092=ADVANCED_FACE('',(#905),#652,.T.);
#5093=ADVANCED_FACE('',(#906,#484),#653,.T.);
#5094=ADVANCED_FACE('',(#907,#485),#654,.F.);
#5220=CLOSED_SHELL('',(#5048,#5049,#5050,#5051,#5052,#5053,#5054,#5055,
#5056,#5057,#5058,#5059,#5060,#5061,#5062,#5063,#5064,#5065,#5066,#5067,
#5068,#5069,#5070,#5071,#5072,#5073,#5074,#5075,#5076,#5077,#5078,#5079,
#5080,#5081,#5082,#5083,#5084,#5085,#5086,#5087,#5088,#5089,#5090,#5091,
#5092,#5093,#5094));
#5811=AXIS2_PLACEMENT_3D('',#8735,#6866,#6867);
#5812=AXIS2_PLACEMENT_3D('',#8736,#6868,#6869);
#5813=AXIS2_PLACEMENT_3D('',#8745,#6874,#6875);
#5814=AXIS2_PLACEMENT_3D('',#8751,#6879,#6880);
#5815=AXIS2_PLACEMENT_3D('',#8757,#6884,#6885);
#5816=AXIS2_PLACEMENT_3D('',#8763,#6889,#6890);
#5817=AXIS2_PLACEMENT_3D('',#8769,#6894,#6895);
#5818=AXIS2_PLACEMENT_3D('',#8775,#6899,#6900);
#5819=AXIS2_PLACEMENT_3D('',#8781,#6904,#6905);
#5820=AXIS2_PLACEMENT_3D('',#8787,#6909,#6910);
#5821=AXIS2_PLACEMENT_3D('',#8793,#6914,#6915);
#5822=AXIS2_PLACEMENT_3D('',#8802,#6920,#6921);
#5823=AXIS2_PLACEMENT_3D('',#8808,#6925,#6926);
#5824=AXIS2_PLACEMENT_3D('',#8814,#6930,#6931);
#5825=AXIS2_PLACEMENT_3D('',#8820,#6935,#6936);
#5826=AXIS2_PLACEMENT_3D('',#8826,#6940,#6941);
#5827=AXIS2_PLACEMENT_3D('',#8832,#6945,#6946);
#5828=AXIS2_PLACEMENT_3D('',#8838,#6950,#6951);
#5829=AXIS2_PLACEMENT_3D('',#8844,#6955,#6956);
#5830=AXIS2_PLACEMENT_3D('',#8850,#6960,#6961);
#5831=AXIS2_PLACEMENT_3D('',#8859,#6966,#6967);
#5832=AXIS2_PLACEMENT_3D('',#8865,#6971,#6972);
#5833=AXIS2_PLACEMENT_3D('',#8871,#6976,#6977);
#5834=AXIS2_PLACEMENT_3D('',#8877,#6981,#6982);
#5835=AXIS2_PLACEMENT_3D('',#8883,#6986,#6987);
#5836=AXIS2_PLACEMENT_3D('',#8889,#6991,#6992);
#5837=AXIS2_PLACEMENT_3D('',#8895,#6996,#6997);
#5838=AXIS2_PLACEMENT_3D('',#8901,#7001,#7002);
#5839=AXIS2_PLACEMENT_3D('',#8907,#7006,#7007);
#5840=AXIS2_PLACEMENT_3D('',#8916,#7012,#7013);
#5841=AXIS2_PLACEMENT_3D('',#8922,#7017,#7018);
#5842=AXIS2_PLACEMENT_3D('',#8928,#7022,#7023);
#5843=AXIS2_PLACEMENT_3D('',#8934,#7027,#7028);
#5844=AXIS2_PLACEMENT_3D('',#8940,#7032,#7033);
#5845=AXIS2_PLACEMENT_3D('',#8946,#7037,#7038);
#5846=AXIS2_PLACEMENT_3D('',#8952,#7042,#7043);
#5847=AXIS2_PLACEMENT_3D('',#8958,#7047,#7048);
#5848=AXIS2_PLACEMENT_3D('',#8964,#7052,#7053);
#5849=AXIS2_PLACEMENT_3D('',#8966,#7054,#7055);
#5850=AXIS2_PLACEMENT_3D('',#8969,#7057,#7058);
#5851=AXIS2_PLACEMENT_3D('',#8970,#7059,#7060);
#5852=AXIS2_PLACEMENT_3D('',#8976,#7064,#7065);
#5853=AXIS2_PLACEMENT_3D('',#8982,#7069,#7070);
#5854=AXIS2_PLACEMENT_3D('',#8985,#7073,#7074);
#5855=AXIS2_PLACEMENT_3D('',#8991,#7078,#7079);
#5856=AXIS2_PLACEMENT_3D('',#8994,#7082,#7083);
#5857=AXIS2_PLACEMENT_3D('',#9000,#7087,#7088);
#5858=AXIS2_PLACEMENT_3D('',#9003,#7091,#7092);
#5859=AXIS2_PLACEMENT_3D('',#9006,#7095,#7096);
#5860=AXIS2_PLACEMENT_3D('',#9007,#7097,#7098);
#6866=DIRECTION('axis',(0.,0.,1.));
#6867=DIRECTION('refdir',(1.,0.,0.));
#6868=DIRECTION('center_axis',(0.,0.,-1.));
#6869=DIRECTION('ref_axis',(0.,1.,0.));
#6870=DIRECTION('',(0.,1.,0.));
#6871=DIRECTION('',(1.,0.,0.));
#6872=DIRECTION('',(0.,-1.,0.));
#6873=DIRECTION('',(1.,0.,0.));
#6874=DIRECTION('center_axis',(0.,1.,-8.88178419700125E-16));
#6875=DIRECTION('ref_axis',(0.,8.88178419700125E-16,1.));
#6876=DIRECTION('',(0.,8.88178419700125E-16,1.));
#6877=DIRECTION('',(1.,0.,0.));
#6878=DIRECTION('',(0.,-8.88178419700125E-16,-1.));
#6879=DIRECTION('center_axis',(0.,-7.40148683083439E-16,-1.));
#6880=DIRECTION('ref_axis',(0.,1.,-7.40148683083439E-16));
#6881=DIRECTION('',(0.,1.,-7.40148683083439E-16));
#6882=DIRECTION('',(1.,0.,0.));
#6883=DIRECTION('',(0.,-1.,7.40148683083439E-16));
#6884=DIRECTION('center_axis',(0.,-0.707106781186547,-0.707106781186548));
#6885=DIRECTION('ref_axis',(0.,0.707106781186548,-0.707106781186547));
#6886=DIRECTION('',(0.,0.707106781186548,-0.707106781186547));
#6887=DIRECTION('',(1.,0.,0.));
#6888=DIRECTION('',(0.,-0.707106781186548,0.707106781186547));
#6889=DIRECTION('center_axis',(0.,-1.,2.77555756156289E-16));
#6890=DIRECTION('ref_axis',(0.,-2.77555756156289E-16,-1.));
#6891=DIRECTION('',(0.,-2.77555756156289E-16,-1.));
#6892=DIRECTION('',(1.,0.,0.));
#6893=DIRECTION('',(0.,2.77555756156289E-16,1.));
#6894=DIRECTION('center_axis',(0.,-0.707106781186547,0.707106781186548));
#6895=DIRECTION('ref_axis',(0.,-0.707106781186548,-0.707106781186547));
#6896=DIRECTION('',(0.,-0.707106781186548,-0.707106781186547));
#6897=DIRECTION('',(1.,0.,0.));
#6898=DIRECTION('',(0.,0.707106781186548,0.707106781186547));
#6899=DIRECTION('center_axis',(0.,7.40148683083438E-16,1.));
#6900=DIRECTION('ref_axis',(0.,-1.,7.40148683083438E-16));
#6901=DIRECTION('',(0.,-1.,7.40148683083438E-16));
#6902=DIRECTION('',(1.,0.,0.));
#6903=DIRECTION('',(0.,1.,-7.40148683083438E-16));
#6904=DIRECTION('center_axis',(0.,1.,-4.44089209850063E-16));
#6905=DIRECTION('ref_axis',(0.,4.44089209850063E-16,1.));
#6906=DIRECTION('',(0.,4.44089209850063E-16,1.));
#6907=DIRECTION('',(1.,0.,0.));
#6908=DIRECTION('',(0.,-4.44089209850063E-16,-1.));
#6909=DIRECTION('center_axis',(0.,2.41352831440251E-16,1.));
#6910=DIRECTION('ref_axis',(0.,-1.,2.41352831440251E-16));
#6911=DIRECTION('',(0.,-1.,2.41352831440251E-16));
#6912=DIRECTION('',(-1.,0.,0.));
#6913=DIRECTION('',(0.,1.,-2.41352831440251E-16));
#6914=DIRECTION('center_axis',(0.,-1.,2.41352831440251E-16));
#6915=DIRECTION('ref_axis',(0.,-2.41352831440251E-16,-1.));
#6916=DIRECTION('',(0.,-2.41352831440251E-16,-1.));
#6917=DIRECTION('',(1.,0.,0.));
#6918=DIRECTION('',(0.,2.41352831440251E-16,1.));
#6919=DIRECTION('',(1.,0.,0.));
#6920=DIRECTION('center_axis',(0.,0.,-1.));
#6921=DIRECTION('ref_axis',(0.,1.,0.));
#6922=DIRECTION('',(0.,1.,0.));
#6923=DIRECTION('',(1.,0.,0.));
#6924=DIRECTION('',(0.,-1.,0.));
#6925=DIRECTION('center_axis',(0.,-1.,0.));
#6926=DIRECTION('ref_axis',(0.,0.,-1.));
#6927=DIRECTION('',(0.,0.,-1.));
#6928=DIRECTION('',(1.,0.,0.));
#6929=DIRECTION('',(0.,0.,1.));
#6930=DIRECTION('center_axis',(0.,-0.707106781186547,0.707106781186548));
#6931=DIRECTION('ref_axis',(0.,-0.707106781186548,-0.707106781186547));
#6932=DIRECTION('',(0.,-0.707106781186548,-0.707106781186547));
#6933=DIRECTION('',(1.,0.,0.));
#6934=DIRECTION('',(0.,0.707106781186548,0.707106781186547));
#6935=DIRECTION('center_axis',(0.,0.,1.));
#6936=DIRECTION('ref_axis',(0.,-1.,0.));
#6937=DIRECTION('',(0.,-1.,0.));
#6938=DIRECTION('',(1.,0.,0.));
#6939=DIRECTION('',(0.,1.,0.));
#6940=DIRECTION('center_axis',(0.,0.707106781186548,0.707106781186547));
#6941=DIRECTION('ref_axis',(0.,-0.707106781186547,0.707106781186548));
#6942=DIRECTION('',(0.,-0.707106781186547,0.707106781186548));
#6943=DIRECTION('',(1.,0.,0.));
#6944=DIRECTION('',(0.,0.707106781186547,-0.707106781186548));
#6945=DIRECTION('center_axis',(0.,1.,0.));
#6946=DIRECTION('ref_axis',(0.,0.,1.));
#6947=DIRECTION('',(0.,0.,1.));
#6948=DIRECTION('',(1.,0.,0.));
#6949=DIRECTION('',(0.,0.,-1.));
#6950=DIRECTION('center_axis',(0.,0.,-1.));
#6951=DIRECTION('ref_axis',(0.,1.,0.));
#6952=DIRECTION('',(0.,1.,0.));
#6953=DIRECTION('',(1.,0.,0.));
#6954=DIRECTION('',(0.,-1.,0.));
#6955=DIRECTION('center_axis',(0.,1.,-2.41352831440251E-16));
#6956=DIRECTION('ref_axis',(0.,2.41352831440251E-16,1.));
#6957=DIRECTION('',(0.,2.41352831440251E-16,1.));
#6958=DIRECTION('',(-1.,0.,0.));
#6959=DIRECTION('',(0.,-2.41352831440251E-16,-1.));
#6960=DIRECTION('center_axis',(0.,0.,1.));
#6961=DIRECTION('ref_axis',(0.,-1.,0.));
#6962=DIRECTION('',(0.,-1.,0.));
#6963=DIRECTION('',(1.,0.,0.));
#6964=DIRECTION('',(0.,1.,0.));
#6965=DIRECTION('',(1.,0.,0.));
#6966=DIRECTION('center_axis',(0.,-1.,0.));
#6967=DIRECTION('ref_axis',(0.,0.,-1.));
#6968=DIRECTION('',(0.,0.,-1.));
#6969=DIRECTION('',(1.,0.,0.));
#6970=DIRECTION('',(0.,0.,1.));
#6971=DIRECTION('center_axis',(0.,0.,1.));
#6972=DIRECTION('ref_axis',(0.,-1.,0.));
#6973=DIRECTION('',(0.,-1.,0.));
#6974=DIRECTION('',(1.,0.,0.));
#6975=DIRECTION('',(0.,1.,0.));
#6976=DIRECTION('center_axis',(0.,0.707106781186548,0.707106781186548));
#6977=DIRECTION('ref_axis',(0.,-0.707106781186548,0.707106781186548));
#6978=DIRECTION('',(0.,-0.707106781186548,0.707106781186548));
#6979=DIRECTION('',(1.,0.,0.));
#6980=DIRECTION('',(0.,0.707106781186548,-0.707106781186548));
#6981=DIRECTION('center_axis',(0.,1.,0.));
#6982=DIRECTION('ref_axis',(0.,0.,1.));
#6983=DIRECTION('',(0.,0.,1.));
#6984=DIRECTION('',(1.,0.,0.));
#6985=DIRECTION('',(0.,0.,-1.));
#6986=DIRECTION('center_axis',(0.,0.707106781186548,-0.707106781186547));
#6987=DIRECTION('ref_axis',(0.,0.707106781186547,0.707106781186548));
#6988=DIRECTION('',(0.,0.707106781186547,0.707106781186548));
#6989=DIRECTION('',(1.,0.,0.));
#6990=DIRECTION('',(0.,-0.707106781186547,-0.707106781186548));
#6991=DIRECTION('center_axis',(0.,-7.40148683083438E-16,-1.));
#6992=DIRECTION('ref_axis',(0.,1.,-7.40148683083438E-16));
#6993=DIRECTION('',(0.,1.,-7.40148683083438E-16));
#6994=DIRECTION('',(1.,0.,0.));
#6995=DIRECTION('',(0.,-1.,7.40148683083438E-16));
#6996=DIRECTION('center_axis',(0.,-1.,0.));
#6997=DIRECTION('ref_axis',(0.,0.,-1.));
#6998=DIRECTION('',(0.,0.,-1.));
#6999=DIRECTION('',(1.,0.,0.));
#7000=DIRECTION('',(0.,0.,1.));
#7001=DIRECTION('center_axis',(0.,0.,-1.));
#7002=DIRECTION('ref_axis',(0.,1.,0.));
#7003=DIRECTION('',(0.,1.,0.));
#7004=DIRECTION('',(-1.,0.,0.));
#7005=DIRECTION('',(0.,-1.,0.));
#7006=DIRECTION('center_axis',(0.,1.,0.));
#7007=DIRECTION('ref_axis',(0.,0.,1.));
#7008=DIRECTION('',(0.,0.,1.));
#7009=DIRECTION('',(1.,0.,0.));
#7010=DIRECTION('',(0.,0.,-1.));
#7011=DIRECTION('',(1.,0.,0.));
#7012=DIRECTION('center_axis',(0.,0.,1.));
#7013=DIRECTION('ref_axis',(0.,-1.,0.));
#7014=DIRECTION('',(0.,-1.,0.));
#7015=DIRECTION('',(1.,0.,0.));
#7016=DIRECTION('',(0.,1.,0.));
#7017=DIRECTION('center_axis',(0.,1.,0.));
#7018=DIRECTION('ref_axis',(0.,0.,1.));
#7019=DIRECTION('',(0.,0.,1.));
#7020=DIRECTION('',(1.,0.,0.));
#7021=DIRECTION('',(0.,0.,-1.));
#7022=DIRECTION('center_axis',(0.,0.707106781186547,-0.707106781186548));
#7023=DIRECTION('ref_axis',(0.,0.707106781186548,0.707106781186547));
#7024=DIRECTION('',(0.,0.707106781186548,0.707106781186547));
#7025=DIRECTION('',(1.,0.,0.));
#7026=DIRECTION('',(0.,-0.707106781186548,-0.707106781186547));
#7027=DIRECTION('center_axis',(0.,0.,-1.));
#7028=DIRECTION('ref_axis',(0.,1.,0.));
#7029=DIRECTION('',(0.,1.,0.));
#7030=DIRECTION('',(1.,0.,0.));
#7031=DIRECTION('',(0.,-1.,0.));
#7032=DIRECTION('center_axis',(0.,-0.707106781186547,-0.707106781186548));
#7033=DIRECTION('ref_axis',(0.,0.707106781186548,-0.707106781186547));
#7034=DIRECTION('',(0.,0.707106781186548,-0.707106781186547));
#7035=DIRECTION('',(1.,0.,0.));
#7036=DIRECTION('',(0.,-0.707106781186548,0.707106781186547));
#7037=DIRECTION('center_axis',(0.,-1.,0.));
#7038=DIRECTION('ref_axis',(0.,0.,-1.));
#7039=DIRECTION('',(0.,0.,-1.));
#7040=DIRECTION('',(1.,0.,0.));
#7041=DIRECTION('',(0.,0.,1.));
#7042=DIRECTION('center_axis',(0.,0.,1.));
#7043=DIRECTION('ref_axis',(0.,-1.,0.));
#7044=DIRECTION('',(0.,-1.,0.));
#7045=DIRECTION('',(1.,0.,0.));
#7046=DIRECTION('',(0.,1.,0.));
#7047=DIRECTION('center_axis',(0.,-1.,0.));
#7048=DIRECTION('ref_axis',(0.,0.,-1.));
#7049=DIRECTION('',(0.,0.,-1.));
#7050=DIRECTION('',(-1.,0.,0.));
#7051=DIRECTION('',(0.,0.,1.));
#7052=DIRECTION('center_axis',(1.,0.,0.));
#7053=DIRECTION('ref_axis',(0.,0.,-1.));
#7054=DIRECTION('center_axis',(1.,0.,0.));
#7055=DIRECTION('ref_axis',(0.,0.,-1.));
#7056=DIRECTION('',(1.,0.,0.));
#7057=DIRECTION('center_axis',(-1.,0.,0.));
#7058=DIRECTION('ref_axis',(0.,0.,-1.));
#7059=DIRECTION('center_axis',(0.,1.,0.));
#7060=DIRECTION('ref_axis',(0.,0.,1.));
#7061=DIRECTION('',(0.,0.,1.));
#7062=DIRECTION('',(1.,0.,0.));
#7063=DIRECTION('',(0.,0.,1.));
#7064=DIRECTION('center_axis',(0.,1.,0.));
#7065=DIRECTION('ref_axis',(0.,0.,1.));
#7066=DIRECTION('',(0.,0.,1.));
#7067=DIRECTION('',(1.,0.,0.));
#7068=DIRECTION('',(0.,0.,1.));
#7069=DIRECTION('center_axis',(0.,0.,-1.));
#7070=DIRECTION('ref_axis',(0.,1.,0.));
#7071=DIRECTION('',(0.,1.,0.));
#7072=DIRECTION('',(0.,1.,0.));
#7073=DIRECTION('center_axis',(0.,0.,-1.));
#7074=DIRECTION('ref_axis',(0.,1.,0.));
#7075=DIRECTION('',(0.,1.,0.));
#7076=DIRECTION('',(1.,0.,0.));
#7077=DIRECTION('',(0.,1.,0.));
#7078=DIRECTION('center_axis',(0.,-1.,0.));
#7079=DIRECTION('ref_axis',(0.,0.,-1.));
#7080=DIRECTION('',(0.,0.,-1.));
#7081=DIRECTION('',(0.,0.,-1.));
#7082=DIRECTION('center_axis',(0.,-1.,0.));
#7083=DIRECTION('ref_axis',(0.,0.,-1.));
#7084=DIRECTION('',(0.,0.,-1.));
#7085=DIRECTION('',(1.,0.,0.));
#7086=DIRECTION('',(0.,0.,-1.));
#7087=DIRECTION('center_axis',(0.,0.,1.));
#7088=DIRECTION('ref_axis',(0.,-1.,0.));
#7089=DIRECTION('',(0.,-1.,0.));
#7090=DIRECTION('',(0.,-1.,0.));
#7091=DIRECTION('center_axis',(0.,0.,1.));
#7092=DIRECTION('ref_axis',(0.,-1.,0.));
#7093=DIRECTION('',(0.,-1.,0.));
#7094=DIRECTION('',(0.,-1.,0.));
#7095=DIRECTION('center_axis',(1.,0.,0.));
#7096=DIRECTION('ref_axis',(0.,0.,-1.));
#7097=DIRECTION('center_axis',(1.,0.,0.));
#7098=DIRECTION('ref_axis',(0.,0.,-1.));
#8735=CARTESIAN_POINT('',(0.,0.,0.));
#8736=CARTESIAN_POINT('Origin',(-0.1,0.82,-0.3));
#8737=CARTESIAN_POINT('',(0.,0.82,-0.3));
#8738=CARTESIAN_POINT('',(0.,1.,-0.3));
#8739=CARTESIAN_POINT('',(0.,0.41,-0.3));
#8740=CARTESIAN_POINT('',(10.,0.82,-0.3));
#8741=CARTESIAN_POINT('',(-0.1,0.82,-0.3));
#8742=CARTESIAN_POINT('',(10.,1.,-0.3));
#8743=CARTESIAN_POINT('',(10.,0.41,-0.3));
#8744=CARTESIAN_POINT('',(-0.05,1.,-0.3));
#8745=CARTESIAN_POINT('Origin',(-0.1,0.82,-0.55));
#8746=CARTESIAN_POINT('',(0.,0.82,-0.55));
#8747=CARTESIAN_POINT('',(0.,0.82,-0.275));
#8748=CARTESIAN_POINT('',(10.,0.82,-0.55));
#8749=CARTESIAN_POINT('',(-0.1,0.82,-0.55));
#8750=CARTESIAN_POINT('',(10.,0.82,-0.275));
#8751=CARTESIAN_POINT('Origin',(-0.1,0.67,-0.55));
#8752=CARTESIAN_POINT('',(0.,0.67,-0.55));
#8753=CARTESIAN_POINT('',(0.,0.335,-0.55));
#8754=CARTESIAN_POINT('',(10.,0.67,-0.55));
#8755=CARTESIAN_POINT('',(-0.1,0.67,-0.55));
#8756=CARTESIAN_POINT('',(10.,0.335,-0.55));
#8757=CARTESIAN_POINT('Origin',(-0.1,0.42,-0.3));
#8758=CARTESIAN_POINT('',(0.,0.42,-0.3));
#8759=CARTESIAN_POINT('',(0.,0.24,-0.12));
#8760=CARTESIAN_POINT('',(10.,0.42,-0.3));
#8761=CARTESIAN_POINT('',(-0.1,0.42,-0.3));
#8762=CARTESIAN_POINT('',(10.,0.24,-0.12));
#8763=CARTESIAN_POINT('Origin',(-0.1,0.42,0.3));
#8764=CARTESIAN_POINT('',(0.,0.42,0.3));
#8765=CARTESIAN_POINT('',(0.,0.42,0.15));
#8766=CARTESIAN_POINT('',(10.,0.42,0.3));
#8767=CARTESIAN_POINT('',(-0.1,0.42,0.3));
#8768=CARTESIAN_POINT('',(10.,0.42,0.15));
#8769=CARTESIAN_POINT('Origin',(-0.1,0.67,0.55));
#8770=CARTESIAN_POINT('',(0.,0.67,0.55));
#8771=CARTESIAN_POINT('',(6.93889390390723E-18,0.365,0.245));
#8772=CARTESIAN_POINT('',(10.,0.67,0.55));
#8773=CARTESIAN_POINT('',(-0.1,0.67,0.55));
#8774=CARTESIAN_POINT('',(10.,0.365,0.245));
#8775=CARTESIAN_POINT('Origin',(-0.1,0.82,0.55));
#8776=CARTESIAN_POINT('',(0.,0.82,0.55));
#8777=CARTESIAN_POINT('',(0.,0.41,0.55));
#8778=CARTESIAN_POINT('',(10.,0.82,0.55));
#8779=CARTESIAN_POINT('',(-0.1,0.82,0.55));
#8780=CARTESIAN_POINT('',(10.,0.41,0.55));
#8781=CARTESIAN_POINT('Origin',(-0.1,0.82,0.3));
#8782=CARTESIAN_POINT('',(0.,0.82,0.3));
#8783=CARTESIAN_POINT('',(0.,0.82,0.15));
#8784=CARTESIAN_POINT('',(10.,0.82,0.3));
#8785=CARTESIAN_POINT('',(-0.1,0.82,0.3));
#8786=CARTESIAN_POINT('',(10.,0.82,0.15));
#8787=CARTESIAN_POINT('Origin',(-0.1,1.05,0.3));
#8788=CARTESIAN_POINT('',(0.,1.,0.3));
#8789=CARTESIAN_POINT('',(0.,0.525,0.3));
#8790=CARTESIAN_POINT('',(10.,1.,0.3));
#8791=CARTESIAN_POINT('',(-0.05,1.,0.3));
#8792=CARTESIAN_POINT('',(10.,0.525,0.3));
#8793=CARTESIAN_POINT('Origin',(-0.1,-0.3,-0.82));
#8794=CARTESIAN_POINT('',(0.,-0.3,-0.82));
#8795=CARTESIAN_POINT('',(0.,-0.3,-1.));
#8796=CARTESIAN_POINT('',(0.,-0.3,-0.41));
#8797=CARTESIAN_POINT('',(10.,-0.3,-0.82));
#8798=CARTESIAN_POINT('',(-0.1,-0.3,-0.82));
#8799=CARTESIAN_POINT('',(10.,-0.3,-1.));
#8800=CARTESIAN_POINT('',(10.,-0.3,-0.41));
#8801=CARTESIAN_POINT('',(-0.05,-0.3,-1.));
#8802=CARTESIAN_POINT('Origin',(-0.1,-0.55,-0.82));
#8803=CARTESIAN_POINT('',(0.,-0.55,-0.82));
#8804=CARTESIAN_POINT('',(0.,-0.275,-0.82));
#8805=CARTESIAN_POINT('',(10.,-0.55,-0.82));
#8806=CARTESIAN_POINT('',(-0.1,-0.55,-0.82));
#8807=CARTESIAN_POINT('',(10.,-0.275,-0.82));
#8808=CARTESIAN_POINT('Origin',(-0.1,-0.55,-0.67));
#8809=CARTESIAN_POINT('',(0.,-0.55,-0.67));
#8810=CARTESIAN_POINT('',(0.,-0.55,-0.335));
#8811=CARTESIAN_POINT('',(10.,-0.55,-0.67));
#8812=CARTESIAN_POINT('',(-0.1,-0.55,-0.67));
#8813=CARTESIAN_POINT('',(10.,-0.55,-0.335));
#8814=CARTESIAN_POINT('Origin',(-0.1,-0.3,-0.42));
#8815=CARTESIAN_POINT('',(0.,-0.3,-0.42));
#8816=CARTESIAN_POINT('',(0.,-0.12,-0.24));
#8817=CARTESIAN_POINT('',(10.,-0.3,-0.42));
#8818=CARTESIAN_POINT('',(-0.1,-0.3,-0.42));
#8819=CARTESIAN_POINT('',(10.,-0.12,-0.24));
#8820=CARTESIAN_POINT('Origin',(-0.1,0.3,-0.42));
#8821=CARTESIAN_POINT('',(0.,0.3,-0.42));
#8822=CARTESIAN_POINT('',(0.,0.15,-0.42));
#8823=CARTESIAN_POINT('',(10.,0.3,-0.42));
#8824=CARTESIAN_POINT('',(-0.1,0.3,-0.42));
#8825=CARTESIAN_POINT('',(10.,0.15,-0.42));
#8826=CARTESIAN_POINT('Origin',(-0.1,0.55,-0.67));
#8827=CARTESIAN_POINT('',(0.,0.55,-0.67));
#8828=CARTESIAN_POINT('',(0.,0.245,-0.365));
#8829=CARTESIAN_POINT('',(10.,0.55,-0.67));
#8830=CARTESIAN_POINT('',(-0.1,0.55,-0.67));
#8831=CARTESIAN_POINT('',(10.,0.245,-0.365));
#8832=CARTESIAN_POINT('Origin',(-0.1,0.55,-0.82));
#8833=CARTESIAN_POINT('',(0.,0.55,-0.82));
#8834=CARTESIAN_POINT('',(0.,0.55,-0.41));
#8835=CARTESIAN_POINT('',(10.,0.55,-0.82));
#8836=CARTESIAN_POINT('',(-0.1,0.55,-0.82));
#8837=CARTESIAN_POINT('',(10.,0.55,-0.41));
#8838=CARTESIAN_POINT('Origin',(-0.1,0.3,-0.82));
#8839=CARTESIAN_POINT('',(0.,0.3,-0.82));
#8840=CARTESIAN_POINT('',(0.,0.15,-0.82));
#8841=CARTESIAN_POINT('',(10.,0.3,-0.82));
#8842=CARTESIAN_POINT('',(-0.1,0.3,-0.82));
#8843=CARTESIAN_POINT('',(10.,0.15,-0.82));
#8844=CARTESIAN_POINT('Origin',(-0.1,0.3,-1.05));
#8845=CARTESIAN_POINT('',(0.,0.3,-1.));
#8846=CARTESIAN_POINT('',(0.,0.3,-0.525));
#8847=CARTESIAN_POINT('',(10.,0.3,-1.));
#8848=CARTESIAN_POINT('',(-0.05,0.3,-1.));
#8849=CARTESIAN_POINT('',(10.,0.3,-0.525));
#8850=CARTESIAN_POINT('Origin',(-0.1,-0.82,0.3));
#8851=CARTESIAN_POINT('',(0.,-0.82,0.3));
#8852=CARTESIAN_POINT('',(0.,-1.,0.3));
#8853=CARTESIAN_POINT('',(0.,-0.41,0.3));
#8854=CARTESIAN_POINT('',(10.,-0.82,0.3));
#8855=CARTESIAN_POINT('',(-0.1,-0.82,0.3));
#8856=CARTESIAN_POINT('',(10.,-1.,0.3));
#8857=CARTESIAN_POINT('',(10.,-0.41,0.3));
#8858=CARTESIAN_POINT('',(-0.05,-1.,0.3));
#8859=CARTESIAN_POINT('Origin',(-0.1,-0.82,0.55));
#8860=CARTESIAN_POINT('',(0.,-0.82,0.55));
#8861=CARTESIAN_POINT('',(0.,-0.82,0.275));
#8862=CARTESIAN_POINT('',(10.,-0.82,0.55));
#8863=CARTESIAN_POINT('',(-0.1,-0.82,0.55));
#8864=CARTESIAN_POINT('',(10.,-0.82,0.275));
#8865=CARTESIAN_POINT('Origin',(-0.1,-0.67,0.55));
#8866=CARTESIAN_POINT('',(0.,-0.67,0.55));
#8867=CARTESIAN_POINT('',(0.,-0.335,0.55));
#8868=CARTESIAN_POINT('',(10.,-0.67,0.55));
#8869=CARTESIAN_POINT('',(-0.1,-0.67,0.55));
#8870=CARTESIAN_POINT('',(10.,-0.335,0.55));
#8871=CARTESIAN_POINT('Origin',(-0.1,-0.42,0.3));
#8872=CARTESIAN_POINT('',(0.,-0.42,0.3));
#8873=CARTESIAN_POINT('',(-6.93889390390723E-18,-0.24,0.12));
#8874=CARTESIAN_POINT('',(10.,-0.42,0.3));
#8875=CARTESIAN_POINT('',(-0.1,-0.42,0.3));
#8876=CARTESIAN_POINT('',(10.,-0.24,0.12));
#8877=CARTESIAN_POINT('Origin',(-0.1,-0.42,-0.3));
#8878=CARTESIAN_POINT('',(0.,-0.42,-0.3));
#8879=CARTESIAN_POINT('',(0.,-0.42,-0.15));
#8880=CARTESIAN_POINT('',(10.,-0.42,-0.3));
#8881=CARTESIAN_POINT('',(-0.1,-0.42,-0.3));
#8882=CARTESIAN_POINT('',(10.,-0.42,-0.15));
#8883=CARTESIAN_POINT('Origin',(-0.1,-0.67,-0.55));
#8884=CARTESIAN_POINT('',(0.,-0.67,-0.55));
#8885=CARTESIAN_POINT('',(0.,-0.365,-0.245));
#8886=CARTESIAN_POINT('',(10.,-0.67,-0.55));
#8887=CARTESIAN_POINT('',(-0.1,-0.67,-0.55));
#8888=CARTESIAN_POINT('',(10.,-0.365,-0.245));
#8889=CARTESIAN_POINT('Origin',(-0.1,-0.82,-0.55));
#8890=CARTESIAN_POINT('',(0.,-0.82,-0.55));
#8891=CARTESIAN_POINT('',(0.,-0.41,-0.55));
#8892=CARTESIAN_POINT('',(10.,-0.82,-0.55));
#8893=CARTESIAN_POINT('',(-0.1,-0.82,-0.55));
#8894=CARTESIAN_POINT('',(10.,-0.41,-0.55));
#8895=CARTESIAN_POINT('Origin',(-0.1,-0.82,-0.3));
#8896=CARTESIAN_POINT('',(0.,-0.82,-0.3));
#8897=CARTESIAN_POINT('',(0.,-0.82,-0.15));
#8898=CARTESIAN_POINT('',(10.,-0.82,-0.3));
#8899=CARTESIAN_POINT('',(-0.1,-0.82,-0.3));
#8900=CARTESIAN_POINT('',(10.,-0.82,-0.15));
#8901=CARTESIAN_POINT('Origin',(-0.1,-1.05,-0.3));
#8902=CARTESIAN_POINT('',(0.,-1.,-0.3));
#8903=CARTESIAN_POINT('',(0.,-0.525,-0.3));
#8904=CARTESIAN_POINT('',(10.,-1.,-0.3));
#8905=CARTESIAN_POINT('',(-0.05,-1.,-0.3));
#8906=CARTESIAN_POINT('',(10.,-0.525,-0.3));
#8907=CARTESIAN_POINT('Origin',(-0.1,0.3,0.82));
#8908=CARTESIAN_POINT('',(0.,0.3,0.82));
#8909=CARTESIAN_POINT('',(0.,0.3,1.));
#8910=CARTESIAN_POINT('',(0.,0.3,0.41));
#8911=CARTESIAN_POINT('',(10.,0.3,0.82));
#8912=CARTESIAN_POINT('',(-0.1,0.3,0.82));
#8913=CARTESIAN_POINT('',(10.,0.3,1.));
#8914=CARTESIAN_POINT('',(10.,0.3,0.41));
#8915=CARTESIAN_POINT('',(-0.05,0.3,1.));
#8916=CARTESIAN_POINT('Origin',(-0.1,0.55,0.82));
#8917=CARTESIAN_POINT('',(0.,0.55,0.82));
#8918=CARTESIAN_POINT('',(0.,0.275,0.82));
#8919=CARTESIAN_POINT('',(10.,0.55,0.82));
#8920=CARTESIAN_POINT('',(-0.1,0.55,0.82));
#8921=CARTESIAN_POINT('',(10.,0.275,0.82));
#8922=CARTESIAN_POINT('Origin',(-0.1,0.55,0.67));
#8923=CARTESIAN_POINT('',(0.,0.55,0.67));
#8924=CARTESIAN_POINT('',(0.,0.55,0.335));
#8925=CARTESIAN_POINT('',(10.,0.55,0.67));
#8926=CARTESIAN_POINT('',(-0.1,0.55,0.67));
#8927=CARTESIAN_POINT('',(10.,0.55,0.335));
#8928=CARTESIAN_POINT('Origin',(-0.1,0.3,0.42));
#8929=CARTESIAN_POINT('',(0.,0.3,0.42));
#8930=CARTESIAN_POINT('',(6.93889390390723E-18,0.12,0.24));
#8931=CARTESIAN_POINT('',(10.,0.3,0.42));
#8932=CARTESIAN_POINT('',(-0.1,0.3,0.42));
#8933=CARTESIAN_POINT('',(10.,0.12,0.24));
#8934=CARTESIAN_POINT('Origin',(-0.1,-0.3,0.42));
#8935=CARTESIAN_POINT('',(0.,-0.3,0.42));
#8936=CARTESIAN_POINT('',(0.,-0.15,0.42));
#8937=CARTESIAN_POINT('',(10.,-0.3,0.42));
#8938=CARTESIAN_POINT('',(-0.1,-0.3,0.42));
#8939=CARTESIAN_POINT('',(10.,-0.15,0.42));
#8940=CARTESIAN_POINT('Origin',(-0.1,-0.55,0.67));
#8941=CARTESIAN_POINT('',(0.,-0.55,0.67));
#8942=CARTESIAN_POINT('',(6.93889390390723E-18,-0.245,0.365));
#8943=CARTESIAN_POINT('',(10.,-0.55,0.67));
#8944=CARTESIAN_POINT('',(-0.1,-0.55,0.67));
#8945=CARTESIAN_POINT('',(10.,-0.245,0.365));
#8946=CARTESIAN_POINT('Origin',(-0.1,-0.55,0.82));
#8947=CARTESIAN_POINT('',(0.,-0.55,0.82));
#8948=CARTESIAN_POINT('',(0.,-0.55,0.41));
#8949=CARTESIAN_POINT('',(10.,-0.55,0.82));
#8950=CARTESIAN_POINT('',(-0.1,-0.55,0.82));
#8951=CARTESIAN_POINT('',(10.,-0.55,0.41));
#8952=CARTESIAN_POINT('Origin',(-0.1,-0.3,0.82));
#8953=CARTESIAN_POINT('',(0.,-0.3,0.82));
#8954=CARTESIAN_POINT('',(0.,-0.15,0.82));
#8955=CARTESIAN_POINT('',(10.,-0.3,0.82));
#8956=CARTESIAN_POINT('',(-0.1,-0.3,0.82));
#8957=CARTESIAN_POINT('',(10.,-0.15,0.82));
#8958=CARTESIAN_POINT('Origin',(-0.1,-0.3,1.05));
#8959=CARTESIAN_POINT('',(0.,-0.3,1.));
#8960=CARTESIAN_POINT('',(0.,-0.3,0.525));
#8961=CARTESIAN_POINT('',(10.,-0.3,1.));
#8962=CARTESIAN_POINT('',(-0.05,-0.3,1.));
#8963=CARTESIAN_POINT('',(10.,-0.3,0.525));
#8964=CARTESIAN_POINT('Origin',(-0.1,0.,0.));
#8965=CARTESIAN_POINT('',(0.,-2.57175827820944E-17,0.21));
#8966=CARTESIAN_POINT('Origin',(0.,0.,0.));
#8967=CARTESIAN_POINT('',(10.,2.57175827820944E-17,0.21));
#8968=CARTESIAN_POINT('',(-0.1,-2.57175827820944E-17,0.21));
#8969=CARTESIAN_POINT('Origin',(10.,0.,0.));
#8970=CARTESIAN_POINT('Origin',(0.,1.,-1.));
#8971=CARTESIAN_POINT('',(0.,1.,1.));
#8972=CARTESIAN_POINT('',(0.,1.,-1.));
#8973=CARTESIAN_POINT('',(10.,1.,1.));
#8974=CARTESIAN_POINT('',(0.,1.,1.));
#8975=CARTESIAN_POINT('',(10.,1.,-1.));
#8976=CARTESIAN_POINT('Origin',(0.,1.,-1.));
#8977=CARTESIAN_POINT('',(10.,1.,-1.));
#8978=CARTESIAN_POINT('',(10.,1.,-1.));
#8979=CARTESIAN_POINT('',(0.,1.,-1.));
#8980=CARTESIAN_POINT('',(0.,1.,-1.));
#8981=CARTESIAN_POINT('',(0.,1.,-1.));
#8982=CARTESIAN_POINT('Origin',(0.,-1.,-1.));
#8983=CARTESIAN_POINT('',(0.,-1.,-1.));
#8984=CARTESIAN_POINT('',(10.,-1.,-1.));
#8985=CARTESIAN_POINT('Origin',(0.,-1.,-1.));
#8986=CARTESIAN_POINT('',(10.,-1.,-1.));
#8987=CARTESIAN_POINT('',(10.,-1.,-1.));
#8988=CARTESIAN_POINT('',(0.,-1.,-1.));
#8989=CARTESIAN_POINT('',(0.,-1.,-1.));
#8990=CARTESIAN_POINT('',(0.,-1.,-1.));
#8991=CARTESIAN_POINT('Origin',(0.,-1.,1.));
#8992=CARTESIAN_POINT('',(0.,-1.,1.));
#8993=CARTESIAN_POINT('',(10.,-1.,1.));
#8994=CARTESIAN_POINT('Origin',(0.,-1.,1.));
#8995=CARTESIAN_POINT('',(10.,-1.,1.));
#8996=CARTESIAN_POINT('',(10.,-1.,1.));
#8997=CARTESIAN_POINT('',(0.,-1.,1.));
#8998=CARTESIAN_POINT('',(0.,-1.,1.));
#8999=CARTESIAN_POINT('',(0.,-1.,1.));
#9000=CARTESIAN_POINT('Origin',(0.,1.,1.));
#9001=CARTESIAN_POINT('',(0.,1.,1.));
#9002=CARTESIAN_POINT('',(10.,1.,1.));
#9003=CARTESIAN_POINT('Origin',(0.,1.,1.));
#9004=CARTESIAN_POINT('',(10.,1.,1.));
#9005=CARTESIAN_POINT('',(0.,1.,1.));
#9006=CARTESIAN_POINT('Origin',(10.,0.,0.));
#9007=CARTESIAN_POINT('Origin',(0.,0.,0.));
#9580=UNCERTAINTY_MEASURE_WITH_UNIT(LENGTH_MEASURE(0.001),#9623,
'DISTANCE_ACCURACY_VALUE',
'Maximum model space distance between geometric entities at asserted c
onnectivities');
#9592=UNCERTAINTY_MEASURE_WITH_UNIT(LENGTH_MEASURE(0.001),#9623,
'DISTANCE_ACCURACY_VALUE',
'Maximum model space distance between geometric entities at asserted c
onnectivities');
#9610=(
GEOMETRIC_REPRESENTATION_CONTEXT(3)
GLOBAL_UNCERTAINTY_ASSIGNED_CONTEXT((#9580))
GLOBAL_UNIT_ASSIGNED_CONTEXT((#9623,#9625,#9626))
REPRESENTATION_CONTEXT('','3D')
);
#9622=(
GEOMETRIC_REPRESENTATION_CONTEXT(3)
GLOBAL_UNCERTAINTY_ASSIGNED_CONTEXT((#9592))
GLOBAL_UNIT_ASSIGNED_CONTEXT((#9623,#9625,#9626))
REPRESENTATION_CONTEXT('','3D')
);
#9623=(
LENGTH_UNIT()
NAMED_UNIT(*)
SI_UNIT(.CENTI.,.METRE.)
);
#9625=(
NAMED_UNIT(*)
PLANE_ANGLE_UNIT()
SI_UNIT($,.RADIAN.)
);
#9626=(
NAMED_UNIT(*)
SI_UNIT($,.STERADIAN.)
SOLID_ANGLE_UNIT()
);
#9644=SHAPE_DEFINITION_REPRESENTATION(#9678,#9761);
#9678=PRODUCT_DEFINITION_SHAPE('',$,#9791);
#9761=SHAPE_REPRESENTATION('',(#5811),#9610);
#9773=PRODUCT_DEFINITION_CONTEXT('part definition',#9862,'design');
#9791=PRODUCT_DEFINITION('Slotted Extrusion - 20 x 20 x 100 mm',
'Slotted Extrusion - 20 x 20 x 100 mm',#9820,#9773);
#9820=PRODUCT_DEFINITION_FORMATION('',$,#9881);
#9862=APPLICATION_CONTEXT(
'Core Data for Automotive Mechanical Design Process');
#9863=PRODUCT_CONTEXT('part definition',#9862,'mechanical');
#9881=PRODUCT('Slotted Extrusion - 20 x 20 x 100 mm',
'Slotted Extrusion - 20 x 20 x 100 mm',
'Slotted Extrusion - 20 x 20 x 100 mm',(#9863));
#9970=COLOUR_RGB('Off White',0.89,0.88,0.83);
#9971=FILL_AREA_STYLE_COLOUR('',#9970);
#9972=FILL_AREA_STYLE('',(#9971));
#9973=SURFACE_STYLE_FILL_AREA(#9972);
#9974=SURFACE_SIDE_STYLE('',(#9973));
#9975=SURFACE_STYLE_USAGE(.BOTH.,#9974);
#9976=PRESENTATION_STYLE_ASSIGNMENT((#9975));
ENDSEC;
END-ISO-10303-21;
